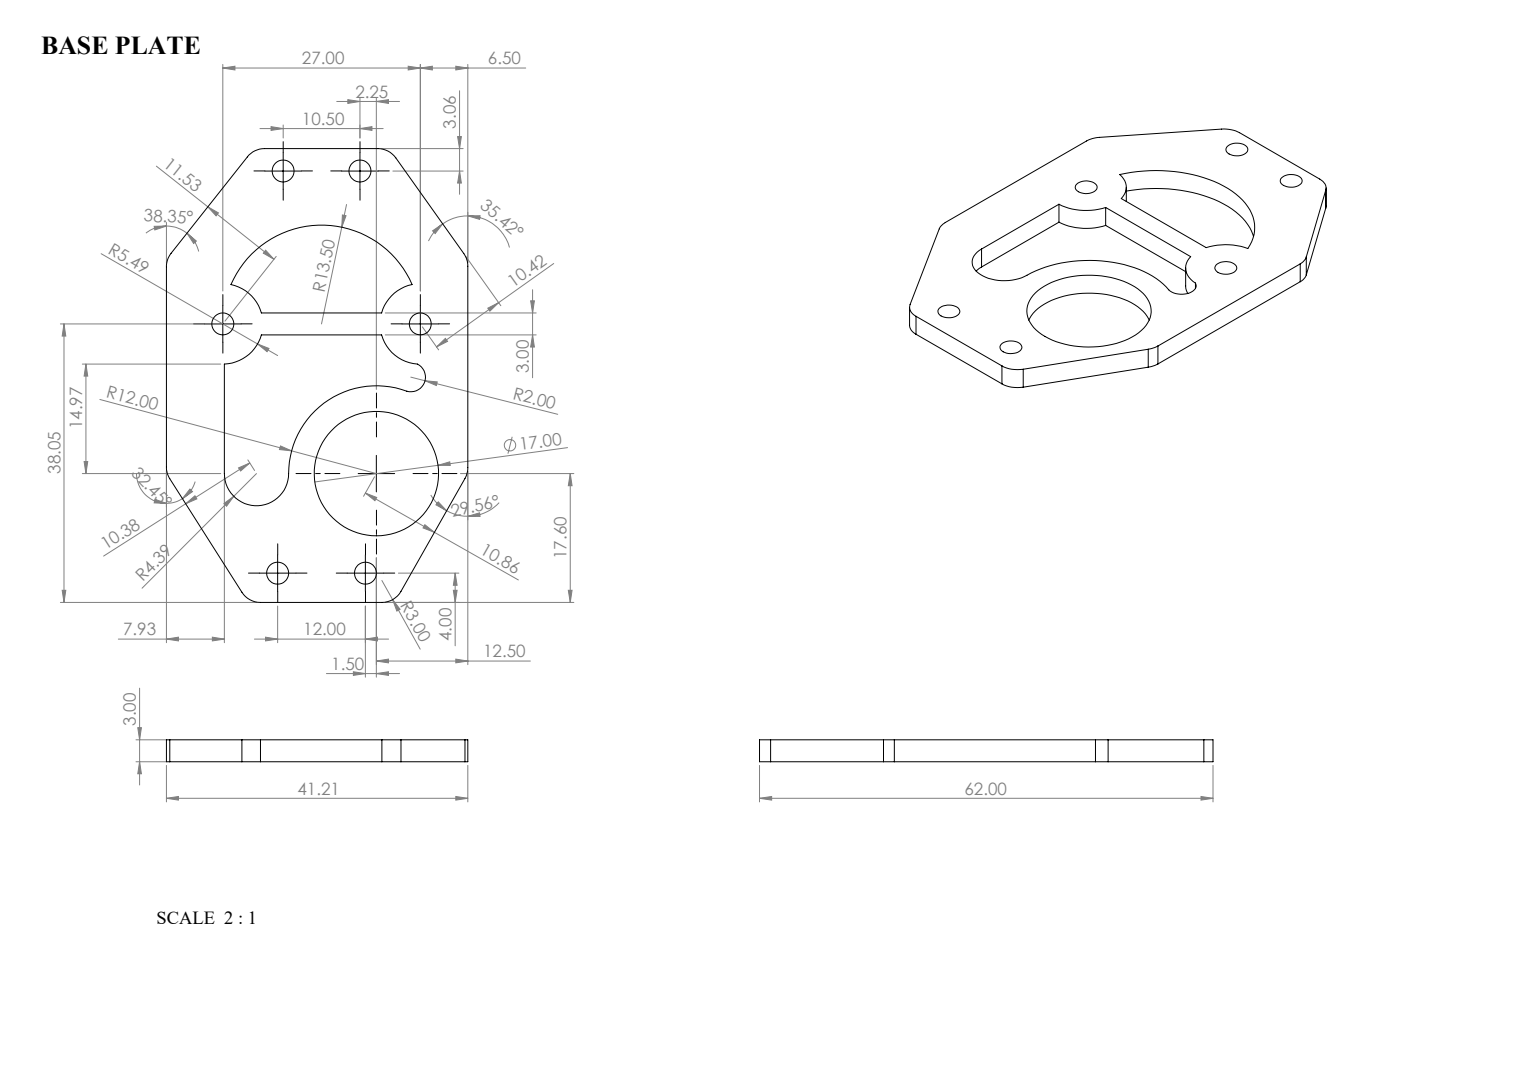
ISO-10303-21;
HEADER;
FILE_DESCRIPTION (('STEP AP214'),
    '1' );
FILE_NAME ('base-plate.step',
    '2026-10-11T23:18:24',
    ( '' ),
    ( '' ),
    'SwSTEP 2.0',
    'SolidWorks 2021',
    '' );
FILE_SCHEMA (( 'AUTOMOTIVE_DESIGN' ));
ENDSEC;

DATA;
#9=FACE_BOUND ( 'NONE', #6807, .T. ) ;
#18=EDGE_LOOP ( 'NONE', ( #222, #3036 ) ) ;
#19=DIRECTION ( 'NONE',  ( -0.000000000000000000, -1.000000000000000000, -0.000000000000000000 ) ) ;
#31=EDGE_CURVE ( 'NONE', #5801, #5272, #8241, .T. ) ;
#45=VERTEX_POINT ( 'NONE', #5075 ) ;
#48=DIRECTION ( 'NONE',  ( 0.000000000000000000, 1.000000000000000000, 0.000000000000000000 ) ) ;
#58=VECTOR ( 'NONE', #8688, 1000.000000000000000 ) ;
#68=VECTOR ( 'NONE', #1053, 1000.000000000000000 ) ;
#77=ORIENTED_EDGE ( 'NONE', *, *, #13230, .T. ) ;
#92=EDGE_CURVE ( 'NONE', #5359, #2558, #6205, .T. ) ;
#98=ORIENTED_EDGE ( 'NONE', *, *, #5069, .T. ) ;
#103=( LENGTH_UNIT ( ) NAMED_UNIT ( * ) SI_UNIT ( .MILLI., .METRE. ) );
#104=DIRECTION ( 'NONE',  ( -0.000000000000000000, -1.000000000000000000, -0.000000000000000000 ) ) ;
#105=CARTESIAN_POINT ( 'NONE',  ( 17.00000000000000711, 0.000000000000000000, 12.57924256039205524 ) ) ;
#107=DIRECTION ( 'NONE',  ( -0.000000000000000000, -1.000000000000000000, -0.000000000000000000 ) ) ;
#111=ADVANCED_FACE ( 'NONE', ( #10454 ), #11355, .F. ) ;
#118=ADVANCED_FACE ( 'NONE', ( #1922 ), #5010, .T. ) ;
#120=CARTESIAN_POINT ( 'NONE',  ( 6.000000000000008882, 3.000000000000000000, 28.50000000000000000 ) ) ;
#124=CARTESIAN_POINT ( 'NONE',  ( -20.74285254778206422, 3.000000000000000000, 14.10762559394868454 ) ) ;
#130=EDGE_CURVE ( 'NONE', #748, #10888, #9495, .T. ) ;
#133=ADVANCED_FACE ( 'NONE', ( #11682 ), #12860, .T. ) ;
#135=ORIENTED_EDGE ( 'NONE', *, *, #11819, .F. ) ;
#147=EDGE_LOOP ( 'NONE', ( #10873, #12283, #1803, #7065 ) ) ;
#148=DIRECTION ( 'NONE',  ( 0.000000000000000000, 1.000000000000000000, 0.000000000000000000 ) ) ;
#150=FACE_BOUND ( 'NONE', #4431, .T. ) ;
#167=DIRECTION ( 'NONE',  ( -1.261435711112880913E-16, -0.000000000000000000, -1.000000000000000000 ) ) ;
#176=CARTESIAN_POINT ( 'NONE',  ( 7.500000000000003553, 0.000000000000000000, 1.399999999999998579 ) ) ;
#180=VERTEX_POINT ( 'NONE', #12788 ) ;
#193=ORIENTED_EDGE ( 'NONE', *, *, #5488, .T. ) ;
#204=ORIENTED_EDGE ( 'NONE', *, *, #9463, .T. ) ;
#208=EDGE_CURVE ( 'NONE', #1513, #12626, #879, .T. ) ;
#222=ORIENTED_EDGE ( 'NONE', *, *, #10239, .T. ) ;
#227=DIRECTION ( 'NONE',  ( 0.000000000000000000, 0.000000000000000000, -1.000000000000000000 ) ) ;
#231=DIRECTION ( 'NONE',  ( -0.000000000000000000, -1.000000000000000000, -0.000000000000000000 ) ) ;
#234=CARTESIAN_POINT ( 'NONE',  ( -20.74285254778206422, 3.000000000000000000, 14.10762559394868454 ) ) ;
#238=ORIENTED_EDGE ( 'NONE', *, *, #208, .T. ) ;
#243=CARTESIAN_POINT ( 'NONE',  ( 7.500000000000003553, 3.000000000000000000, 13.39999999999999858 ) ) ;
#247=CIRCLE ( 'NONE', #1345, 13.50000000000000178 ) ;
#253=AXIS2_PLACEMENT_3D ( 'NONE', #1336, #11952, #4576 ) ;
#265=CARTESIAN_POINT ( 'NONE',  ( -7.798201703419555209, 3.000000000000000000, -30.99999999999999289 ) ) ;
#280=CARTESIAN_POINT ( 'NONE',  ( -21.21140389626389577, 3.000000000000000000, -14.83930531255814955 ) ) ;
#287=ORIENTED_EDGE ( 'NONE', *, *, #2381, .F. ) ;
#308=ORIENTED_EDGE ( 'NONE', *, *, #11057, .T. ) ;
#314=DIRECTION ( 'NONE',  ( -0.000000000000000000, -1.000000000000000000, -0.000000000000000000 ) ) ;
#330=DIRECTION ( 'NONE',  ( -0.000000000000000000, -1.000000000000000000, -0.000000000000000000 ) ) ;
#361=ORIENTED_EDGE ( 'NONE', *, *, #12415, .F. ) ;
#371=DIRECTION ( 'NONE',  ( 0.000000000000000000, 0.000000000000000000, 1.000000000000000000 ) ) ;
#375=VERTEX_POINT ( 'NONE', #9174 ) ;
#381=CARTESIAN_POINT ( 'NONE',  ( 12.21000000000000796, 3.000000000000000000, 0.2208617994340217328 ) ) ;
#383=DIRECTION ( 'NONE',  ( 0.000000000000000000, 0.000000000000000000, -1.000000000000000000 ) ) ;
#415=LINE ( 'NONE', #13021, #10839 ) ;
#435=CARTESIAN_POINT ( 'NONE',  ( 20.00000000000000711, 0.000000000000000000, 12.57924256039204280 ) ) ;
#447=VERTEX_POINT ( 'NONE', #8333 ) ;
#452=CIRCLE ( 'NONE', #7929, 5.499999999999996447 ) ;
#457=LINE ( 'NONE', #7759, #5366 ) ;
#463=CIRCLE ( 'NONE', #3104, 5.486375544325371223 ) ;
#469=ORIENTED_EDGE ( 'NONE', *, *, #9034, .T. ) ;
#470=LINE ( 'NONE', #8726, #4829 ) ;
#471=VECTOR ( 'NONE', #5300, 1000.000000000000000 ) ;
#472=CARTESIAN_POINT ( 'NONE',  ( 12.21000000000000796, 3.000000000000000000, 0.2208617994340217328 ) ) ;
#477=ORIENTED_EDGE ( 'NONE', *, *, #3906, .F. ) ;
#480=UNCERTAINTY_MEASURE_WITH_UNIT (LENGTH_MEASURE( 1.000000000000000082E-05 ), #13297, 'distance_accuracy_value', 'NONE');
#485=ORIENTED_EDGE ( 'NONE', *, *, #6813, .T. ) ;
#497=ORIENTED_EDGE ( 'NONE', *, *, #9087, .T. ) ;
#503=AXIS2_PLACEMENT_3D ( 'NONE', #11418, #6309, #4045 ) ;
#506=CARTESIAN_POINT ( 'NONE',  ( -13.49999999999999645, 0.000000000000000000, -8.549999999999998934 ) ) ;
#526=DIRECTION ( 'NONE',  ( -0.000000000000000000, -1.000000000000000000, -0.000000000000000000 ) ) ;
#528=PRODUCT ( 'base-plate', 'base-plate', '', ( #2121 ) ) ;
#554=DIRECTION ( 'NONE',  ( 1.269138026879196405E-16, 0.000000000000000000, 1.000000000000000000 ) ) ;
#560=AXIS2_PLACEMENT_3D ( 'NONE', #3107, #4208, #10695 ) ;
#577=ORIENTED_EDGE ( 'NONE', *, *, #13185, .F. ) ;
#583=CARTESIAN_POINT ( 'NONE',  ( 8.252687871541644071, 0.000000000000000000, 28.00000000000000000 ) ) ;
#585=DIRECTION ( 'NONE',  ( 0.000000000000000000, 0.000000000000000000, 1.000000000000000000 ) ) ;
#595=EDGE_LOOP ( 'NONE', ( #4853, #1217, #4392, #497, #6612, #11542, #2963, #3783 ) ) ;
#598=CARTESIAN_POINT ( 'NONE',  ( -21.21140389626389222, 0.000000000000000000, 12.49772878833445056 ) ) ;
#607=EDGE_CURVE ( 'NONE', #10071, #5801, #415, .T. ) ;
#621=DIRECTION ( 'NONE',  ( 0.000000000000000000, 0.000000000000000000, 1.000000000000000000 ) ) ;
#634=CARTESIAN_POINT ( 'NONE',  ( -12.38517345876401521, 3.000000000000000000, -12.42191571009144901 ) ) ;
#660=FACE_OUTER_BOUND ( 'NONE', #10677, .T. ) ;
#675=ORIENTED_EDGE ( 'NONE', *, *, #4510, .T. ) ;
#681=EDGE_CURVE ( 'NONE', #2253, #3491, #9506, .T. ) ;
#704=DIRECTION ( 'NONE',  ( 0.000000000000000000, 0.000000000000000000, -1.000000000000000000 ) ) ;
#705=ORIENTED_EDGE ( 'NONE', *, *, #2472, .T. ) ;
#716=CIRCLE ( 'NONE', #13481, 5.486375544325371223 ) ;
#724=PLANE ( 'NONE',  #1129 ) ;
#725=CYLINDRICAL_SURFACE ( 'NONE', #10420, 2.999999999999999112 ) ;
#726=CYLINDRICAL_SURFACE ( 'NONE', #3574, 1.500000000000001332 ) ;
#732=VERTEX_POINT ( 'NONE', #2758 ) ;
#748=VERTEX_POINT ( 'NONE', #8122 ) ;
#779=CARTESIAN_POINT ( 'NONE',  ( -13.49999999999999645, 0.000000000000000000, -7.049999999999998934 ) ) ;
#802=DIRECTION ( 'NONE',  ( -0.000000000000000000, -1.000000000000000000, -0.000000000000000000 ) ) ;
#811=LINE ( 'NONE', #5002, #9521 ) ;
#812=CARTESIAN_POINT ( 'NONE',  ( 7.500000000000003553, 3.000000000000000000, 4.899999999999997691 ) ) ;
#828=ORIENTED_EDGE ( 'NONE', *, *, #11819, .T. ) ;
#833=VERTEX_POINT ( 'NONE', #12065 ) ;
#834=DIRECTION ( 'NONE',  ( 0.000000000000000000, 1.000000000000000000, -0.000000000000000000 ) ) ;
#840=CARTESIAN_POINT ( 'NONE',  ( 8.252687871541644071, 3.000000000000000000, 28.00000000000000000 ) ) ;
#851=PLANE ( 'NONE',  #4516 ) ;
#852=CARTESIAN_POINT ( 'NONE',  ( 8.208497377870827449, 3.000000000000000000, -8.550000000000002487 ) ) ;
#853=CARTESIAN_POINT ( 'NONE',  ( -5.999999999999991118, 0.000000000000000000, 28.50000000000000000 ) ) ;
#867=ORIENTED_EDGE ( 'NONE', *, *, #6355, .F. ) ;
#870=CARTESIAN_POINT ( 'NONE',  ( 7.702138240596505092, 3.000000000000000000, -30.99999999999999289 ) ) ;
#877=ORIENTED_EDGE ( 'NONE', *, *, #6306, .T. ) ;
#879=LINE ( 'NONE', #11884, #4882 ) ;
#889=CARTESIAN_POINT ( 'NONE',  ( -7.798201703419567643, 3.000000000000000000, -27.99999999999999289 ) ) ;
#894=VECTOR ( 'NONE', #3788, 1000.000000000000000 ) ;
#906=DIRECTION ( 'NONE',  ( 0.000000000000000000, 1.000000000000000000, 0.000000000000000000 ) ) ;
#907=DIRECTION ( 'NONE',  ( 0.000000000000000000, 0.000000000000000000, 1.000000000000000000 ) ) ;
#909=EDGE_LOOP ( 'NONE', ( #5022, #6085, #12147, #4456 ) ) ;
#923=CYLINDRICAL_SURFACE ( 'NONE', #4474, 1.499999999999997780 ) ;
#930=VERTEX_POINT ( 'NONE', #3159 ) ;
#932=ORIENTED_EDGE ( 'NONE', *, *, #8564, .T. ) ;
#936=EDGE_CURVE ( 'NONE', #7585, #7204, #7318, .T. ) ;
#950=ORIENTED_EDGE ( 'NONE', *, *, #13438, .T. ) ;
#962=AXIS2_PLACEMENT_3D ( 'NONE', #3139, #7989, #12209 ) ;
#975=CARTESIAN_POINT ( 'NONE',  ( 3.469446951953614189E-15, 0.000000000000000000, -20.55000000000000071 ) ) ;
#983=AXIS2_PLACEMENT_3D ( 'NONE', #6603, #5774, #12198 ) ;
#991=LINE ( 'NONE', #852, #68 ) ;
#996=CIRCLE ( 'NONE', #4722, 1.500000000000001332 ) ;
#998=VECTOR ( 'NONE', #2423, 1000.000000000000114 ) ;
#1005=ORIENTED_EDGE ( 'NONE', *, *, #10913, .T. ) ;
#1042=DIRECTION ( 'NONE',  ( 0.000000000000000000, 1.000000000000000000, -0.000000000000000000 ) ) ;
#1053=DIRECTION ( 'NONE',  ( -0.000000000000000000, -1.000000000000000000, -0.000000000000000000 ) ) ;
#1070=CARTESIAN_POINT ( 'NONE',  ( 5.250000000000000000, 0.000000000000000000, -27.94078293894052578 ) ) ;
#1077=DIRECTION ( 'NONE',  ( -0.000000000000000000, -1.000000000000000000, -0.000000000000000000 ) ) ;
#1080=ADVANCED_FACE ( 'NONE', ( #4393 ), #6669, .T. ) ;
#1081=CARTESIAN_POINT ( 'NONE',  ( 6.000000000000008882, 3.000000000000000000, 25.50000000000000000 ) ) ;
#1087=DIRECTION ( 'NONE',  ( -1.000000000000000000, -0.000000000000000000, -0.000000000000000000 ) ) ;
#1106=FACE_OUTER_BOUND ( 'NONE', #909, .T. ) ;
#1115=EDGE_CURVE ( 'NONE', #3649, #2964, #8630, .T. ) ;
#1122=EDGE_CURVE ( 'NONE', #4943, #748, #7568, .T. ) ;
#1129=AXIS2_PLACEMENT_3D ( 'NONE', #6919, #2580, #11188 ) ;
#1130=CIRCLE ( 'NONE', #7717, 2.000000000000000444 ) ;
#1137=AXIS2_PLACEMENT_3D ( 'NONE', #10482, #6075, #10412 ) ;
#1151=DIRECTION ( 'NONE',  ( -0.000000000000000000, -1.000000000000000000, -0.000000000000000000 ) ) ;
#1163=CARTESIAN_POINT ( 'NONE',  ( -13.49999999999999645, 3.000000000000000000, -7.049999999999998934 ) ) ;
#1166=ORIENTED_EDGE ( 'NONE', *, *, #5988, .F. ) ;
#1167=FACE_BOUND ( 'NONE', #595, .T. ) ;
#1171=AXIS2_PLACEMENT_3D ( 'NONE', #3827, #4855, #8029 ) ;
#1189=AXIS2_PLACEMENT_3D ( 'NONE', #12887, #3430, #7642 ) ;
#1191=CARTESIAN_POINT ( 'NONE',  ( -5.999999999999991118, 3.000000000000000000, 27.00000000000000000 ) ) ;
#1199=DIRECTION ( 'NONE',  ( -0.5795187626277481518, -0.000000000000000000, -0.8149588969772669778 ) ) ;
#1204=ORIENTED_EDGE ( 'NONE', *, *, #12712, .F. ) ;
#1217=ORIENTED_EDGE ( 'NONE', *, *, #12857, .T. ) ;
#1220=DIRECTION ( 'NONE',  ( 0.000000000000000000, 1.000000000000000000, 0.000000000000000000 ) ) ;
#1232=ORIENTED_EDGE ( 'NONE', *, *, #4731, .T. ) ;
#1251=VERTEX_POINT ( 'NONE', #6946 ) ;
#1257=CARTESIAN_POINT ( 'NONE',  ( 13.50000000000000355, 3.000000000000000000, -7.050000000000000711 ) ) ;
#1260=DIRECTION ( 'NONE',  ( 0.000000000000000000, 1.000000000000000000, 0.000000000000000000 ) ) ;
#1280=VERTEX_POINT ( 'NONE', #11075 ) ;
#1283=FACE_OUTER_BOUND ( 'NONE', #7951, .T. ) ;
#1289=CARTESIAN_POINT ( 'NONE',  ( -12.38517345876401521, 0.000000000000000000, -12.42191571009144901 ) ) ;
#1295=CARTESIAN_POINT ( 'NONE',  ( -8.352599575481690408, 3.000000000000000000, 28.00000000000000000 ) ) ;
#1303=ADVANCED_FACE ( 'NONE', ( #6243 ), #5149, .T. ) ;
#1317=LINE ( 'NONE', #9588, #12455 ) ;
#1318=CIRCLE ( 'NONE', #2016, 1.500000000000001332 ) ;
#1320=DIRECTION ( 'NONE',  ( -0.000000000000000000, -1.000000000000000000, -0.000000000000000000 ) ) ;
#1335=DIRECTION ( 'NONE',  ( -0.000000000000000000, -1.000000000000000000, -0.000000000000000000 ) ) ;
#1336=CARTESIAN_POINT ( 'NONE',  ( -13.49999999999999645, 3.000000000000000000, -7.049999999999998934 ) ) ;
#1345=AXIS2_PLACEMENT_3D ( 'NONE', #7820, #3415, #10926 ) ;
#1363=CARTESIAN_POINT ( 'NONE',  ( -7.798201703419567643, 3.000000000000000000, -27.99999999999999289 ) ) ;
#1364=ORIENTED_EDGE ( 'NONE', *, *, #9776, .F. ) ;
#1380=AXIS2_PLACEMENT_3D ( 'NONE', #2769, #13035, #1743 ) ;
#1390=( NAMED_UNIT ( * ) PLANE_ANGLE_UNIT ( ) SI_UNIT ( $, .RADIAN. ) );
#1398=LINE ( 'NONE', #234, #998 ) ;
#1403=ADVANCED_FACE ( 'NONE', ( #3137 ), #3672, .T. ) ;
#1409=VERTEX_POINT ( 'NONE', #12093 ) ;
#1410=DIRECTION ( 'NONE',  ( 0.000000000000000000, 1.000000000000000000, 0.000000000000000000 ) ) ;
#1422=CIRCLE ( 'NONE', #5602, 4.390701948131951582 ) ;
#1454=( NAMED_UNIT ( * ) SI_UNIT ( $, .STERADIAN. ) SOLID_ANGLE_UNIT ( ) );
#1457=PRODUCT_DEFINITION_CONTEXT ( 'detailed design', #12167, 'design' ) ;
#1465=ADVANCED_FACE ( 'NONE', ( #5950 ), #13260, .F. ) ;
#1470=ORIENTED_EDGE ( 'NONE', *, *, #8368, .T. ) ;
#1479=DIRECTION ( 'NONE',  ( -0.000000000000000000, -1.000000000000000000, -0.000000000000000000 ) ) ;
#1489=DIRECTION ( 'NONE',  ( -0.6204948238377417935, -0.000000000000000000, 0.7842105416216806901 ) ) ;
#1503=ADVANCED_FACE ( 'NONE', ( #2924 ), #725, .T. ) ;
#1505=CYLINDRICAL_SURFACE ( 'NONE', #12322, 1.499999999999999556 ) ;
#1507=CARTESIAN_POINT ( 'NONE',  ( 20.00000000000000711, 3.000000000000000000, 12.57924256039204280 ) ) ;
#1513=VERTEX_POINT ( 'NONE', #6993 ) ;
#1515=VERTEX_POINT ( 'NONE', #7874 ) ;
#1532=CYLINDRICAL_SURFACE ( 'NONE', #6265, 1.500000000000001332 ) ;
#1549=FACE_BOUND ( 'NONE', #2100, .T. ) ;
#1550=CARTESIAN_POINT ( 'NONE',  ( 5.250000000000000000, 3.000000000000000000, -27.94078293894052578 ) ) ;
#1559=DIRECTION ( 'NONE',  ( 0.000000000000000000, 1.000000000000000000, 0.000000000000000000 ) ) ;
#1567=ORIENTED_EDGE ( 'NONE', *, *, #11702, .F. ) ;
#1600=CIRCLE ( 'NONE', #7756, 2.999999999999999112 ) ;
#1612=AXIS2_PLACEMENT_3D ( 'NONE', #5175, #8323, #10405 ) ;
#1613=AXIS2_PLACEMENT_3D ( 'NONE', #13583, #19, #10548 ) ;
#1614=DIRECTION ( 'NONE',  ( 0.000000000000000000, 0.000000000000000000, -1.000000000000000000 ) ) ;
#1622=FACE_BOUND ( 'NONE', #4217, .T. ) ;
#1626=AXIS2_PLACEMENT_3D ( 'NONE', #11875, #9668, #5531 ) ;
#1629=ADVANCED_FACE ( 'NONE', ( #3784 ), #8372, .F. ) ;
#1631=EDGE_CURVE ( 'NONE', #8075, #1251, #9534, .T. ) ;
#1642=DIRECTION ( 'NONE',  ( -1.000000000000000000, -0.000000000000000000, 1.055752450943286591E-16 ) ) ;
#1664=AXIS2_PLACEMENT_3D ( 'NONE', #2975, #7186, #11378 ) ;
#1668=VERTEX_POINT ( 'NONE', #3475 ) ;
#1678=FACE_OUTER_BOUND ( 'NONE', #5525, .T. ) ;
#1684=PRODUCT_DEFINITION_FORMATION_WITH_SPECIFIED_SOURCE ( 'ANY', '', #528, .NOT_KNOWN. ) ;
#1694=CARTESIAN_POINT ( 'NONE',  ( 3.469446951953614189E-15, 3.000000000000000000, -7.049999999999999822 ) ) ;
#1700=CARTESIAN_POINT ( 'NONE',  ( -21.21140389626389577, 3.000000000000000000, -14.83930531255815133 ) ) ;
#1714=VERTEX_POINT ( 'NONE', #4380 ) ;
#1729=UNCERTAINTY_MEASURE_WITH_UNIT (LENGTH_MEASURE( 1.000000000000000082E-05 ), #103, 'distance_accuracy_value', 'NONE');
#1736=VERTEX_POINT ( 'NONE', #3413 ) ;
#1742=VERTEX_POINT ( 'NONE', #5543 ) ;
#1743=DIRECTION ( 'NONE',  ( 0.000000000000000000, 0.000000000000000000, -1.000000000000000000 ) ) ;
#1755=DIRECTION ( 'NONE',  ( 0.000000000000000000, 0.000000000000000000, 1.000000000000000000 ) ) ;
#1802=CIRCLE ( 'NONE', #253, 1.499999999999998668 ) ;
#1803=ORIENTED_EDGE ( 'NONE', *, *, #11372, .F. ) ;
#1806=FACE_OUTER_BOUND ( 'NONE', #13472, .T. ) ;
#1811=AXIS2_PLACEMENT_3D ( 'NONE', #10518, #1077, #13417 ) ;
#1813=AXIS2_PLACEMENT_3D ( 'NONE', #12705, #3315, #5319 ) ;
#1829=EDGE_CURVE ( 'NONE', #5704, #11250, #10986, .T. ) ;
#1831=CARTESIAN_POINT ( 'NONE',  ( -13.49999999999999645, 3.000000000000000000, -7.049999999999998934 ) ) ;
#1834=ORIENTED_EDGE ( 'NONE', *, *, #10278, .T. ) ;
#1838=VERTEX_POINT ( 'NONE', #598 ) ;
#1845=DIRECTION ( 'NONE',  ( 0.000000000000000000, 0.000000000000000000, 1.000000000000000000 ) ) ;
#1859=AXIS2_PLACEMENT_3D ( 'NONE', #3543, #10859, #2450 ) ;
#1881=ADVANCED_FACE ( 'NONE', ( #10159 ), #10089, .T. ) ;
#1910=EDGE_CURVE ( 'NONE', #1668, #1714, #12249, .T. ) ;
#1919=CARTESIAN_POINT ( 'NONE',  ( -13.28140389626389783, 0.000000000000000000, 13.39999999999999858 ) ) ;
#1922=FACE_OUTER_BOUND ( 'NONE', #3038, .T. ) ;
#1926=DIRECTION ( 'NONE',  ( -0.000000000000000000, -1.000000000000000000, -0.000000000000000000 ) ) ;
#1928=DIRECTION ( 'NONE',  ( -0.000000000000000000, -1.000000000000000000, -0.000000000000000000 ) ) ;
#1934=ORIENTED_EDGE ( 'NONE', *, *, #3335, .T. ) ;
#1957=DIRECTION ( 'NONE',  ( -0.000000000000000000, -1.000000000000000000, -0.000000000000000000 ) ) ;
#1969=EDGE_CURVE ( 'NONE', #8365, #12893, #8158, .T. ) ;
#1977=VECTOR ( 'NONE', #1151, 1000.000000000000000 ) ;
#1978=DIRECTION ( 'NONE',  ( -0.000000000000000000, -1.000000000000000000, -0.000000000000000000 ) ) ;
#1980=ORIENTED_EDGE ( 'NONE', *, *, #13096, .F. ) ;
#1989=DIRECTION ( 'NONE',  ( -0.000000000000000000, -1.000000000000000000, -0.000000000000000000 ) ) ;
#2000=ORIENTED_EDGE ( 'NONE', *, *, #2363, .T. ) ;
#2002=VECTOR ( 'NONE', #2219, 1000.000000000000000 ) ;
#2005=CIRCLE ( 'NONE', #10360, 5.486375544325371223 ) ;
#2008=LINE ( 'NONE', #6202, #3327 ) ;
#2016=AXIS2_PLACEMENT_3D ( 'NONE', #3607, #2438, #8760 ) ;
#2022=EDGE_CURVE ( 'NONE', #4834, #8240, #9329, .T. ) ;
#2029=VERTEX_POINT ( 'NONE', #13547 ) ;
#2033=VERTEX_POINT ( 'NONE', #12583 ) ;
#2034=AXIS2_PLACEMENT_3D ( 'NONE', #3071, #7284, #11481 ) ;
#2046=AXIS2_PLACEMENT_3D ( 'NONE', #3810, #13115, #585 ) ;
#2047=EDGE_CURVE ( 'NONE', #5599, #2682, #12427, .T. ) ;
#2051=ORIENTED_EDGE ( 'NONE', *, *, #3303, .F. ) ;
#2060=EDGE_CURVE ( 'NONE', #930, #13159, #3377, .T. ) ;
#2073=FACE_BOUND ( 'NONE', #18, .T. ) ;
#2100=EDGE_LOOP ( 'NONE', ( #2226, #8679 ) ) ;
#2103=AXIS2_PLACEMENT_3D ( 'NONE', #9001, #13218, #13089 ) ;
#2107=DIRECTION ( 'NONE',  ( 0.8438162171727213723, 0.000000000000000000, -0.5366322685380732205 ) ) ;
#2108=CARTESIAN_POINT ( 'NONE',  ( 12.37962962962963864, 3.000000000000000000, -12.43467921358330663 ) ) ;
#2121=PRODUCT_CONTEXT ( 'NONE', #8884, 'mechanical' ) ;
#2122=DIRECTION ( 'NONE',  ( -0.000000000000000000, -1.000000000000000000, -0.000000000000000000 ) ) ;
#2137=CARTESIAN_POINT ( 'NONE',  ( 13.50000000000000355, 0.000000000000000000, -5.550000000000001599 ) ) ;
#2145=EDGE_CURVE ( 'NONE', #6080, #1742, #5459, .T. ) ;
#2150=EDGE_CURVE ( 'NONE', #3649, #5599, #3256, .T. ) ;
#2151=PLANE ( 'NONE',  #2311 ) ;
#2153=CARTESIAN_POINT ( 'NONE',  ( 13.50000000000000355, 0.000000000000000000, -7.050000000000000711 ) ) ;
#2154=LINE ( 'NONE', #5315, #7062 ) ;
#2163=EDGE_CURVE ( 'NONE', #10097, #12683, #11083, .T. ) ;
#2168=DIRECTION ( 'NONE',  ( 0.000000000000000000, 0.000000000000000000, 1.000000000000000000 ) ) ;
#2176=ORIENTED_EDGE ( 'NONE', *, *, #10005, .T. ) ;
#2190=ORIENTED_EDGE ( 'NONE', *, *, #6830, .T. ) ;
#2193=CARTESIAN_POINT ( 'NONE',  ( -8.352599575481690408, 3.000000000000000000, 30.99999999999999289 ) ) ;
#2212=VERTEX_POINT ( 'NONE', #435 ) ;
#2218=DIRECTION ( 'NONE',  ( 0.000000000000000000, 0.000000000000000000, 1.000000000000000000 ) ) ;
#2219=DIRECTION ( 'NONE',  ( -0.000000000000000000, -1.000000000000000000, -0.000000000000000000 ) ) ;
#2226=ORIENTED_EDGE ( 'NONE', *, *, #10278, .F. ) ;
#2233=PLANE ( 'NONE',  #13273 ) ;
#2253=VERTEX_POINT ( 'NONE', #506 ) ;
#2258=VECTOR ( 'NONE', #7072, 1000.000000000000000 ) ;
#2282=CIRCLE ( 'NONE', #10203, 1.500000000000001332 ) ;
#2283=EDGE_CURVE ( 'NONE', #10892, #10734, #2720, .T. ) ;
#2294=ORIENTED_EDGE ( 'NONE', *, *, #8948, .F. ) ;
#2304=EDGE_CURVE ( 'NONE', #11250, #6484, #11758, .T. ) ;
#2309=CARTESIAN_POINT ( 'NONE',  ( -8.890701948131944476, 0.000000000000000000, 13.39999999999999858 ) ) ;
#2311=AXIS2_PLACEMENT_3D ( 'NONE', #5383, #11724, #2356 ) ;
#2314=CARTESIAN_POINT ( 'NONE',  ( -8.222660081691577361, 0.000000000000000000, -8.549999999999998934 ) ) ;
#2316=ORIENTED_EDGE ( 'NONE', *, *, #6450, .F. ) ;
#2337=ORIENTED_EDGE ( 'NONE', *, *, #9364, .F. ) ;
#2349=VERTEX_POINT ( 'NONE', #12371 ) ;
#2356=DIRECTION ( 'NONE',  ( -1.000000000000000000, 0.000000000000000000, -0.000000000000000000 ) ) ;
#2358=LINE ( 'NONE', #5447, #6645 ) ;
#2363=EDGE_CURVE ( 'NONE', #375, #2349, #3043, .T. ) ;
#2370=VERTEX_POINT ( 'NONE', #6087 ) ;
#2371=ORIENTED_EDGE ( 'NONE', *, *, #10453, .F. ) ;
#2381=EDGE_CURVE ( 'NONE', #3023, #4625, #13086, .T. ) ;
#2382=CARTESIAN_POINT ( 'NONE',  ( 8.252687871541644071, 3.000000000000000000, 28.00000000000000000 ) ) ;
#2386=CYLINDRICAL_SURFACE ( 'NONE', #12106, 4.390701948131951582 ) ;
#2396=ORIENTED_EDGE ( 'NONE', *, *, #7136, .T. ) ;
#2397=VERTEX_POINT ( 'NONE', #12564 ) ;
#2400=DIRECTION ( 'NONE',  ( -0.000000000000000000, -1.000000000000000000, -0.000000000000000000 ) ) ;
#2404=PLANE ( 'NONE',  #983 ) ;
#2408=ORIENTED_EDGE ( 'NONE', *, *, #9087, .F. ) ;
#2417=CIRCLE ( 'NONE', #10989, 5.499999999999996447 ) ;
#2418=DIRECTION ( 'NONE',  ( -0.000000000000000000, -1.000000000000000000, -0.000000000000000000 ) ) ;
#2420=AXIS2_PLACEMENT_3D ( 'NONE', #2918, #9592, #5385 ) ;
#2423=DIRECTION ( 'NONE',  ( 0.5366322685380732205, 0.000000000000000000, 0.8438162171727212613 ) ) ;
#2425=CARTESIAN_POINT ( 'NONE',  ( 10.14701493152832512, 0.000000000000000000, -29.73855628788322747 ) ) ;
#2428=CIRCLE ( 'NONE', #2860, 1.500000000000001332 ) ;
#2438=DIRECTION ( 'NONE',  ( 0.000000000000000000, 1.000000000000000000, 0.000000000000000000 ) ) ;
#2442=EDGE_LOOP ( 'NONE', ( #1232, #11128, #3557, #3779 ) ) ;
#2443=ORIENTED_EDGE ( 'NONE', *, *, #12580, .F. ) ;
#2445=AXIS2_PLACEMENT_3D ( 'NONE', #9870, #7615, #6573 ) ;
#2450=DIRECTION ( 'NONE',  ( 1.000000000000000000, 0.000000000000000000, -0.000000000000000000 ) ) ;
#2454=LINE ( 'NONE', #812, #9672 ) ;
#2463=ORIENTED_EDGE ( 'NONE', *, *, #1910, .T. ) ;
#2464=CARTESIAN_POINT ( 'NONE',  ( 12.37962962962963864, 3.000000000000000000, -12.43467921358330663 ) ) ;
#2472=EDGE_CURVE ( 'NONE', #3370, #11639, #1317, .T. ) ;
#2482=CARTESIAN_POINT ( 'NONE',  ( -13.49999999999999645, 0.000000000000000000, -7.049999999999998934 ) ) ;
#2487=CARTESIAN_POINT ( 'NONE',  ( -8.352599575481690408, 0.000000000000000000, 30.99999999999999289 ) ) ;
#2489=FILL_AREA_STYLE ('',( #4555 ) ) ;
#2490=CIRCLE ( 'NONE', #1626, 1.499999999999998668 ) ;
#2492=DIRECTION ( 'NONE',  ( 0.000000000000000000, 1.000000000000000000, -0.000000000000000000 ) ) ;
#2509=CIRCLE ( 'NONE', #8877, 12.00000000000000000 ) ;
#2515=ORIENTED_EDGE ( 'NONE', *, *, #2163, .T. ) ;
#2517=ORIENTED_EDGE ( 'NONE', *, *, #6588, .T. ) ;
#2527=STYLED_ITEM ( 'NONE', ( #7719 ), #3745 ) ;
#2529=CIRCLE ( 'NONE', #8674, 1.500000000000001332 ) ;
#2530=ADVANCED_FACE ( 'NONE', ( #11596 ), #2151, .F. ) ;
#2542=DIRECTION ( 'NONE',  ( -0.000000000000000000, -1.000000000000000000, -0.000000000000000000 ) ) ;
#2558=VERTEX_POINT ( 'NONE', #10693 ) ;
#2580=DIRECTION ( 'NONE',  ( 0.000000000000000000, -1.000000000000000000, 0.000000000000000000 ) ) ;
#2614=ORIENTED_EDGE ( 'NONE', *, *, #2304, .T. ) ;
#2623=AXIS2_PLACEMENT_3D ( 'NONE', #3492, #10800, #11910 ) ;
#2629=ORIENTED_EDGE ( 'NONE', *, *, #7346, .F. ) ;
#2634=CARTESIAN_POINT ( 'NONE',  ( -8.890701948131944476, 3.000000000000000000, 13.39999999999999858 ) ) ;
#2655=CARTESIAN_POINT ( 'NONE',  ( -20.56403552112892896, 3.000000000000000000, -16.70078978407140013 ) ) ;
#2660=AXIS2_PLACEMENT_3D ( 'NONE', #9121, #8907, #11125 ) ;
#2661=ORIENTED_EDGE ( 'NONE', *, *, #2022, .T. ) ;
#2682=VERTEX_POINT ( 'NONE', #2487 ) ;
#2684=ORIENTED_EDGE ( 'NONE', *, *, #2047, .T. ) ;
#2696=ORIENTED_EDGE ( 'NONE', *, *, #3385, .T. ) ;
#2707=DIRECTION ( 'NONE',  ( 0.000000000000000000, 0.000000000000000000, -1.000000000000000000 ) ) ;
#2712=FACE_BOUND ( 'NONE', #10036, .T. ) ;
#2720=CIRCLE ( 'NONE', #5368, 13.50000000000000178 ) ;
#2734=VECTOR ( 'NONE', #1978, 1000.000000000000000 ) ;
#2744=AXIS2_PLACEMENT_3D ( 'NONE', #13045, #3525, #3664 ) ;
#2752=EDGE_CURVE ( 'NONE', #4632, #5256, #3472, .T. ) ;
#2758=CARTESIAN_POINT ( 'NONE',  ( -7.798201703419555209, 0.000000000000000000, -30.99999999999999289 ) ) ;
#2760=CARTESIAN_POINT ( 'NONE',  ( 7.500000000000003553, 0.000000000000000000, 13.39999999999999858 ) ) ;
#2769=CARTESIAN_POINT ( 'NONE',  ( -13.49999999999999645, 3.000000000000000000, -7.049999999999998934 ) ) ;
#2789=ORIENTED_EDGE ( 'NONE', *, *, #1829, .F. ) ;
#2800=CARTESIAN_POINT ( 'NONE',  ( 19.44487669093179605, 3.000000000000000000, -16.66326752702930847 ) ) ;
#2815=LINE ( 'NONE', #11015, #5780 ) ;
#2835=ORIENTED_EDGE ( 'NONE', *, *, #9258, .T. ) ;
#2860=AXIS2_PLACEMENT_3D ( 'NONE', #11334, #13183, #13336 ) ;
#2901=FACE_OUTER_BOUND ( 'NONE', #7066, .T. ) ;
#2908=ADVANCED_FACE ( 'NONE', ( #12743, #1167, #6393, #150, #4399, #8460, #9, #12685, #2073, #5294 ), #7571, .T. ) ;
#2912=CARTESIAN_POINT ( 'NONE',  ( -20.74285254778206067, 3.000000000000000000, 14.10762559394868099 ) ) ;
#2914=CARTESIAN_POINT ( 'NONE',  ( -5.999999999999991118, 0.000000000000000000, 27.00000000000000000 ) ) ;
#2918=CARTESIAN_POINT ( 'NONE',  ( -13.28140389626389783, 3.000000000000000000, 13.39999999999999858 ) ) ;
#2924=FACE_OUTER_BOUND ( 'NONE', #13436, .T. ) ;
#2932=DIRECTION ( 'NONE',  ( -0.000000000000000000, -1.000000000000000000, -0.000000000000000000 ) ) ;
#2940=DIRECTION ( 'NONE',  ( -0.000000000000000000, -1.000000000000000000, -0.000000000000000000 ) ) ;
#2963=ORIENTED_EDGE ( 'NONE', *, *, #13274, .T. ) ;
#2964=VERTEX_POINT ( 'NONE', #2193 ) ;
#2975=CARTESIAN_POINT ( 'NONE',  ( 17.00000000000000711, 3.000000000000000000, 12.57924256039205524 ) ) ;
#2989=CARTESIAN_POINT ( 'NONE',  ( -20.74285254778206422, 0.000000000000000000, 14.10762559394868454 ) ) ;
#2991=LINE ( 'NONE', #11395, #5277 ) ;
#3009=DIRECTION ( 'NONE',  ( 0.000000000000000000, 0.000000000000000000, -1.000000000000000000 ) ) ;
#3021=CARTESIAN_POINT ( 'NONE',  ( 13.50000000000000355, 3.000000000000000000, -5.550000000000001599 ) ) ;
#3023=VERTEX_POINT ( 'NONE', #3161 ) ;
#3028=PRODUCT_DEFINITION ( 'UNKNOWN', '', #1684, #1457 ) ;
#3035=CARTESIAN_POINT ( 'NONE',  ( -5.999999999999991118, 0.000000000000000000, 27.00000000000000000 ) ) ;
#3036=ORIENTED_EDGE ( 'NONE', *, *, #10962, .T. ) ;
#3038=EDGE_LOOP ( 'NONE', ( #11382, #2337, #10364, #5538 ) ) ;
#3041=EDGE_CURVE ( 'NONE', #2033, #12313, #8992, .T. ) ;
#3043=LINE ( 'NONE', #2912, #3168 ) ;
#3047=DIRECTION ( 'NONE',  ( 0.5366322685380732205, 0.000000000000000000, 0.8438162171727212613 ) ) ;
#3048=CARTESIAN_POINT ( 'NONE',  ( 7.702138240596516638, 3.000000000000000000, -27.99999999999999289 ) ) ;
#3059=ADVANCED_FACE ( 'NONE', ( #6601 ), #1505, .F. ) ;
#3062=DIRECTION ( 'NONE',  ( 0.000000000000000000, 0.000000000000000000, 1.000000000000000000 ) ) ;
#3067=DIRECTION ( 'NONE',  ( 0.000000000000000000, 1.000000000000000000, -0.000000000000000000 ) ) ;
#3069=EDGE_LOOP ( 'NONE', ( #8602, #1980, #6687, #5840 ) ) ;
#3070=EDGE_CURVE ( 'NONE', #2033, #8075, #470, .T. ) ;
#3071=CARTESIAN_POINT ( 'NONE',  ( -5.250000000000000000, 3.000000000000000000, -27.94078293894052578 ) ) ;
#3082=AXIS2_PLACEMENT_3D ( 'NONE', #3360, #3227, #6536 ) ;
#3095=CARTESIAN_POINT ( 'NONE',  ( 3.469446951953614189E-15, 3.000000000000000000, -20.55000000000000071 ) ) ;
#3098=ADVANCED_FACE ( 'NONE', ( #5491 ), #9699, .T. ) ;
#3104=AXIS2_PLACEMENT_3D ( 'NONE', #8100, #11272, #1845 ) ;
#3107=CARTESIAN_POINT ( 'NONE',  ( -21.21140389626389577, 3.000000000000000000, -14.83930531255815133 ) ) ;
#3108=DIRECTION ( 'NONE',  ( -0.000000000000000000, -1.000000000000000000, -0.000000000000000000 ) ) ;
#3109=DIRECTION ( 'NONE',  ( 0.000000000000000000, 1.000000000000000000, 0.000000000000000000 ) ) ;
#3122=AXIS2_PLACEMENT_3D ( 'NONE', #11280, #12531, #7157 ) ;
#3123=AXIS2_PLACEMENT_3D ( 'NONE', #9612, #7674, #383 ) ;
#3131=VECTOR ( 'NONE', #5384, 1000.000000000000000 ) ;
#3137=FACE_OUTER_BOUND ( 'NONE', #11415, .T. ) ;
#3139=CARTESIAN_POINT ( 'NONE',  ( 5.250000000000000000, 3.000000000000000000, -27.94078293894052578 ) ) ;
#3140=PRODUCT_DEFINITION_SHAPE ( 'NONE', 'NONE',  #3028 ) ;
#3143=CARTESIAN_POINT ( 'NONE',  ( 20.00000000000000711, 3.000000000000000000, 12.57924256039204280 ) ) ;
#3156=ORIENTED_EDGE ( 'NONE', *, *, #7047, .T. ) ;
#3159=CARTESIAN_POINT ( 'NONE',  ( 10.14701493152832512, 0.000000000000000000, -29.73855628788322747 ) ) ;
#3161=CARTESIAN_POINT ( 'NONE',  ( 5.250000000000000000, 3.000000000000000000, -26.44078293894052578 ) ) ;
#3168=VECTOR ( 'NONE', #5041, 1000.000000000000000 ) ;
#3176=VECTOR ( 'NONE', #8703, 1000.000000000000000 ) ;
#3178=CIRCLE ( 'NONE', #6255, 2.999999999999999112 ) ;
#3188=MECHANICAL_DESIGN_GEOMETRIC_PRESENTATION_REPRESENTATION('',(#2527),#4076);
#3197=ORIENTED_EDGE ( 'NONE', *, *, #3974, .F. ) ;
#3205=DIRECTION ( 'NONE',  ( 0.000000000000000000, 0.000000000000000000, 1.000000000000000000 ) ) ;
#3206=CARTESIAN_POINT ( 'NONE',  ( 17.00000000000000355, 3.000000000000000000, -14.92471123914605435 ) ) ;
#3219=CARTESIAN_POINT ( 'NONE',  ( -8.222660081691577361, 3.000000000000000000, -5.549999999999999822 ) ) ;
#3227=DIRECTION ( 'NONE',  ( 0.000000000000000000, -1.000000000000000000, 0.000000000000000000 ) ) ;
#3243=ORIENTED_EDGE ( 'NONE', *, *, #9776, .T. ) ;
#3246=DIRECTION ( 'NONE',  ( 0.000000000000000000, 1.000000000000000000, 0.000000000000000000 ) ) ;
#3256=LINE ( 'NONE', #4433, #13060 ) ;
#3260=CARTESIAN_POINT ( 'NONE',  ( 10.86210944460165528, 0.000000000000000000, 29.48017534571043541 ) ) ;
#3289=DIRECTION ( 'NONE',  ( 0.000000000000000000, 1.000000000000000000, 0.000000000000000000 ) ) ;
#3294=AXIS2_PLACEMENT_3D ( 'NONE', #9701, #10681, #10539 ) ;
#3296=EDGE_LOOP ( 'NONE', ( #6577, #5303, #675, #4112 ) ) ;
#3303=EDGE_CURVE ( 'NONE', #5027, #3357, #5081, .T. ) ;
#3315=DIRECTION ( 'NONE',  ( -0.000000000000000000, -1.000000000000000000, -0.000000000000000000 ) ) ;
#3319=CARTESIAN_POINT ( 'NONE',  ( 5.250000000000000000, 3.000000000000000000, -29.44078293894052933 ) ) ;
#3327=VECTOR ( 'NONE', #12359, 1000.000000000000000 ) ;
#3330=CARTESIAN_POINT ( 'NONE',  ( -8.222660081691577361, 3.000000000000000000, -8.549999999999998934 ) ) ;
#3335=EDGE_CURVE ( 'NONE', #12461, #4201, #6313, .T. ) ;
#3356=AXIS2_PLACEMENT_3D ( 'NONE', #12930, #7625, #9752 ) ;
#3357=VERTEX_POINT ( 'NONE', #5351 ) ;
#3360=CARTESIAN_POINT ( 'NONE',  ( -7.798201703419567643, 0.000000000000000000, -27.99999999999999289 ) ) ;
#3370=VERTEX_POINT ( 'NONE', #3143 ) ;
#3377=CIRCLE ( 'NONE', #4701, 2.999999999999999112 ) ;
#3378=AXIS2_PLACEMENT_3D ( 'NONE', #7576, #6542, #6474 ) ;
#3381=DIRECTION ( 'NONE',  ( 0.000000000000000000, 0.000000000000000000, 1.000000000000000000 ) ) ;
#3382=FACE_OUTER_BOUND ( 'NONE', #7189, .T. ) ;
#3383=CYLINDRICAL_SURFACE ( 'NONE', #7697, 8.500000000000000000 ) ;
#3385=EDGE_CURVE ( 'NONE', #13469, #45, #8507, .T. ) ;
#3391=EDGE_LOOP ( 'NONE', ( #12627, #12308, #1470, #238 ) ) ;
#3399=AXIS2_PLACEMENT_3D ( 'NONE', #7040, #13239, #5796 ) ;
#3402=DIRECTION ( 'NONE',  ( 0.000000000000000000, 0.000000000000000000, 1.000000000000000000 ) ) ;
#3408=VECTOR ( 'NONE', #9978, 1000.000000000000000 ) ;
#3409=ORIENTED_EDGE ( 'NONE', *, *, #11372, .T. ) ;
#3413=CARTESIAN_POINT ( 'NONE',  ( -10.15083332828461771, 3.000000000000000000, -29.86148447151320795 ) ) ;
#3414=FACE_OUTER_BOUND ( 'NONE', #7967, .T. ) ;
#3415=DIRECTION ( 'NONE',  ( 0.000000000000000000, 1.000000000000000000, 0.000000000000000000 ) ) ;
#3417=CARTESIAN_POINT ( 'NONE',  ( -7.798201703419567643, 0.000000000000000000, -27.99999999999999289 ) ) ;
#3422=EDGE_LOOP ( 'NONE', ( #1567, #287 ) ) ;
#3430=DIRECTION ( 'NONE',  ( 0.000000000000000000, 1.000000000000000000, 0.000000000000000000 ) ) ;
#3456=EDGE_LOOP ( 'NONE', ( #11445, #7984, #6228, #8705 ) ) ;
#3462=DIRECTION ( 'NONE',  ( 0.000000000000000000, 0.000000000000000000, 1.000000000000000000 ) ) ;
#3470=ORIENTED_EDGE ( 'NONE', *, *, #9513, .F. ) ;
#3472=CIRCLE ( 'NONE', #8104, 2.999999999999999112 ) ;
#3475=CARTESIAN_POINT ( 'NONE',  ( -21.21140389626389577, 3.000000000000000000, -14.83930531255814955 ) ) ;
#3491=VERTEX_POINT ( 'NONE', #12232 ) ;
#3492=CARTESIAN_POINT ( 'NONE',  ( 7.500000000000003553, 3.000000000000000000, 13.39999999999999858 ) ) ;
#3510=DIRECTION ( 'NONE',  ( 0.000000000000000000, 0.000000000000000000, 1.000000000000000000 ) ) ;
#3518=LINE ( 'NONE', #2425, #5115 ) ;
#3520=ORIENTED_EDGE ( 'NONE', *, *, #13438, .F. ) ;
#3521=VECTOR ( 'NONE', #5004, 1000.000000000000000 ) ;
#3525=DIRECTION ( 'NONE',  ( -0.000000000000000000, -1.000000000000000000, -0.000000000000000000 ) ) ;
#3540=VECTOR ( 'NONE', #10293, 1000.000000000000000 ) ;
#3543=CARTESIAN_POINT ( 'NONE',  ( -7.798201703419555209, 3.000000000000000000, -30.99999999999999289 ) ) ;
#3544=ADVANCED_FACE ( 'NONE', ( #1283 ), #5545, .T. ) ;
#3552=CARTESIAN_POINT ( 'NONE',  ( 3.469446951953614189E-15, 3.000000000000000000, -7.049999999999999822 ) ) ;
#3557=ORIENTED_EDGE ( 'NONE', *, *, #130, .F. ) ;
#3560=AXIS2_PLACEMENT_3D ( 'NONE', #2482, #9842, #6551 ) ;
#3569=CARTESIAN_POINT ( 'NONE',  ( 13.11311062740304401, 3.000000000000000000, -1.563624455674628377 ) ) ;
#3572=FACE_OUTER_BOUND ( 'NONE', #8262, .T. ) ;
#3574=AXIS2_PLACEMENT_3D ( 'NONE', #1550, #12166, #5741 ) ;
#3607=CARTESIAN_POINT ( 'NONE',  ( 6.000000000000008882, 0.000000000000000000, 27.00000000000000000 ) ) ;
#3613=ADVANCED_FACE ( 'NONE', ( #3414 ), #2386, .F. ) ;
#3622=AXIS2_PLACEMENT_3D ( 'NONE', #7393, #12759, #227 ) ;
#3634=EDGE_CURVE ( 'NONE', #10193, #7606, #6808, .T. ) ;
#3649=VERTEX_POINT ( 'NONE', #7257 ) ;
#3664=DIRECTION ( 'NONE',  ( 0.000000000000000000, 0.000000000000000000, 1.000000000000000000 ) ) ;
#3672=PLANE ( 'NONE',  #9747 ) ;
#3683=ADVANCED_FACE ( 'NONE', ( #5117 ), #7197, .T. ) ;
#3686=LINE ( 'NONE', #6789, #13503 ) ;
#3689=ORIENTED_EDGE ( 'NONE', *, *, #7911, .T. ) ;
#3692=DIRECTION ( 'NONE',  ( 0.000000000000000000, 0.000000000000000000, 1.000000000000000000 ) ) ;
#3702=VERTEX_POINT ( 'NONE', #853 ) ;
#3707=ORIENTED_EDGE ( 'NONE', *, *, #6449, .F. ) ;
#3733=ADVANCED_FACE ( 'NONE', ( #3940 ), #8143, .T. ) ;
#3745=ADVANCED_BREP_SHAPE_REPRESENTATION ( '', ( #8567, #10007 ), #10678 ) ;
#3763=ORIENTED_EDGE ( 'NONE', *, *, #10239, .F. ) ;
#3768=CIRCLE ( 'NONE', #1137, 12.00000000000000000 ) ;
#3779=ORIENTED_EDGE ( 'NONE', *, *, #1122, .F. ) ;
#3783=ORIENTED_EDGE ( 'NONE', *, *, #10040, .T. ) ;
#3784=FACE_OUTER_BOUND ( 'NONE', #6403, .T. ) ;
#3788=DIRECTION ( 'NONE',  ( -0.000000000000000000, -1.000000000000000000, -0.000000000000000000 ) ) ;
#3791=VECTOR ( 'NONE', #3047, 1000.000000000000114 ) ;
#3792=VECTOR ( 'NONE', #10358, 1000.000000000000000 ) ;
#3808=DIRECTION ( 'NONE',  ( 0.000000000000000000, 0.000000000000000000, 1.000000000000000000 ) ) ;
#3810=CARTESIAN_POINT ( 'NONE',  ( 12.21000000000000796, 0.000000000000000000, 0.2208617994340217328 ) ) ;
#3815=CYLINDRICAL_SURFACE ( 'NONE', #4205, 1.499999999999999556 ) ;
#3818=CARTESIAN_POINT ( 'NONE',  ( -8.222660081691577361, 3.000000000000000000, -8.549999999999998934 ) ) ;
#3820=AXIS2_PLACEMENT_3D ( 'NONE', #243, #8825, #3402 ) ;
#3824=ADVANCED_FACE ( 'NONE', ( #4356 ), #3383, .F. ) ;
#3827=CARTESIAN_POINT ( 'NONE',  ( 17.00000000000000355, 3.000000000000000000, -14.92471123914605435 ) ) ;
#3830=DIRECTION ( 'NONE',  ( -0.000000000000000000, -0.000000000000000000, 1.000000000000000000 ) ) ;
#3834=DIRECTION ( 'NONE',  ( -0.000000000000000000, -1.000000000000000000, -0.000000000000000000 ) ) ;
#3836=CARTESIAN_POINT ( 'NONE',  ( 20.00000000000000355, 0.000000000000000000, -14.92471123914604370 ) ) ;
#3838=ORIENTED_EDGE ( 'NONE', *, *, #607, .F. ) ;
#3852=FACE_OUTER_BOUND ( 'NONE', #6929, .T. ) ;
#3884=EDGE_LOOP ( 'NONE', ( #3470, #13020, #5382, #13016 ) ) ;
#3886=EDGE_LOOP ( 'NONE', ( #1834, #8435, #4979, #13296 ) ) ;
#3893=EDGE_CURVE ( 'NONE', #6080, #13469, #13207, .T. ) ;
#3901=CARTESIAN_POINT ( 'NONE',  ( 19.60942157306000766, 3.000000000000000000, 14.05941790610251374 ) ) ;
#3906=EDGE_CURVE ( 'NONE', #11282, #4803, #2154, .T. ) ;
#3909=EDGE_CURVE ( 'NONE', #5272, #2212, #12357, .T. ) ;
#3937=DIRECTION ( 'NONE',  ( 0.000000000000000000, 1.000000000000000000, 0.000000000000000000 ) ) ;
#3940=FACE_OUTER_BOUND ( 'NONE', #6664, .T. ) ;
#3946=DIRECTION ( 'NONE',  ( -1.000000000000000000, 0.000000000000000000, -0.000000000000000000 ) ) ;
#3955=CARTESIAN_POINT ( 'NONE',  ( 7.500000000000003553, 0.000000000000000000, 13.39999999999999858 ) ) ;
#3972=ORIENTED_EDGE ( 'NONE', *, *, #8368, .F. ) ;
#3974=EDGE_CURVE ( 'NONE', #1409, #732, #10896, .T. ) ;
#3999=AXIS2_PLACEMENT_3D ( 'NONE', #2382, #6578, #6517 ) ;
#4030=ORIENTED_EDGE ( 'NONE', *, *, #8822, .F. ) ;
#4033=VECTOR ( 'NONE', #526, 1000.000000000000000 ) ;
#4037=CARTESIAN_POINT ( 'NONE',  ( 7.500000000000003553, 0.000000000000000000, 4.899999999999997691 ) ) ;
#4044=AXIS2_PLACEMENT_3D ( 'NONE', #13404, #7212, #3062 ) ;
#4045=DIRECTION ( 'NONE',  ( 0.000000000000000000, 0.000000000000000000, -1.000000000000000000 ) ) ;
#4076=( GEOMETRIC_REPRESENTATION_CONTEXT ( 3 ) GLOBAL_UNCERTAINTY_ASSIGNED_CONTEXT ( ( #10811 ) ) GLOBAL_UNIT_ASSIGNED_CONTEXT ( ( #11858, #1390, #6555 ) ) REPRESENTATION_CONTEXT ( 'NONE', 'WORKASPACE' ) );
#4082=ADVANCED_FACE ( 'NONE', ( #1806 ), #6001, .F. ) ;
#4086=CARTESIAN_POINT ( 'NONE',  ( 6.000000000000008882, 3.000000000000000000, 25.50000000000000000 ) ) ;
#4112=ORIENTED_EDGE ( 'NONE', *, *, #10962, .F. ) ;
#4118=LINE ( 'NONE', #3219, #9468 ) ;
#4128=EDGE_CURVE ( 'NONE', #10071, #6484, #7575, .T. ) ;
#4139=VERTEX_POINT ( 'NONE', #8664 ) ;
#4163=CARTESIAN_POINT ( 'NONE',  ( 7.702138240596505092, 0.000000000000000000, -30.99999999999999289 ) ) ;
#4186=VECTOR ( 'NONE', #10479, 1000.000000000000000 ) ;
#4201=VERTEX_POINT ( 'NONE', #2137 ) ;
#4205=AXIS2_PLACEMENT_3D ( 'NONE', #1831, #10150, #7809 ) ;
#4206=EDGE_LOOP ( 'NONE', ( #9644, #8816, #4374, #8749, #8121, #13546, #10810, #5937, #4312, #12062, #6715, #4488, #12878, #7693, #11634, #12361 ) ) ;
#4208=DIRECTION ( 'NONE',  ( 1.000000000000000000, 0.000000000000000000, -1.269138026879196405E-16 ) ) ;
#4217=EDGE_LOOP ( 'NONE', ( #12111, #7925 ) ) ;
#4237=CIRCLE ( 'NONE', #3356, 3.000000000000002665 ) ;
#4253=EDGE_CURVE ( 'NONE', #9985, #11282, #8159, .T. ) ;
#4263=EDGE_LOOP ( 'NONE', ( #7861, #7877, #13073, #8192, #8962 ) ) ;
#4265=VECTOR ( 'NONE', #3834, 1000.000000000000000 ) ;
#4275=DIRECTION ( 'NONE',  ( -0.000000000000000000, -0.000000000000000000, 1.000000000000000000 ) ) ;
#4276=ORIENTED_EDGE ( 'NONE', *, *, #9463, .F. ) ;
#4280=VECTOR ( 'NONE', #1928, 1000.000000000000000 ) ;
#4295=ORIENTED_EDGE ( 'NONE', *, *, #11702, .T. ) ;
#4305=EDGE_CURVE ( 'NONE', #3370, #2212, #5846, .T. ) ;
#4312=ORIENTED_EDGE ( 'NONE', *, *, #2304, .F. ) ;
#4321=EDGE_CURVE ( 'NONE', #12313, #833, #1130, .T. ) ;
#4335=ORIENTED_EDGE ( 'NONE', *, *, #13266, .F. ) ;
#4355=CYLINDRICAL_SURFACE ( 'NONE', #11275, 1.500000000000001332 ) ;
#4356=FACE_OUTER_BOUND ( 'NONE', #3886, .T. ) ;
#4357=LINE ( 'NONE', #4420, #2002 ) ;
#4374=ORIENTED_EDGE ( 'NONE', *, *, #2060, .F. ) ;
#4380=CARTESIAN_POINT ( 'NONE',  ( -21.21140389626389222, 3.000000000000000000, 12.49772878833445056 ) ) ;
#4392=ORIENTED_EDGE ( 'NONE', *, *, #1631, .T. ) ;
#4393=FACE_OUTER_BOUND ( 'NONE', #147, .T. ) ;
#4399=FACE_OUTER_BOUND ( 'NONE', #4206, .T. ) ;
#4410=EDGE_CURVE ( 'NONE', #5397, #1515, #2005, .T. ) ;
#4420=CARTESIAN_POINT ( 'NONE',  ( 20.00000000000000355, 3.000000000000000000, -14.92471123914604370 ) ) ;
#4426=CIRCLE ( 'NONE', #9263, 2.999999999999999112 ) ;
#4429=ORIENTED_EDGE ( 'NONE', *, *, #7588, .F. ) ;
#4431=EDGE_LOOP ( 'NONE', ( #2661, #13080 ) ) ;
#4433=CARTESIAN_POINT ( 'NONE',  ( -10.88404822699983576, 3.000000000000000000, 29.60989680561421622 ) ) ;
#4434=LINE ( 'NONE', #6709, #13304 ) ;
#4448=CIRCLE ( 'NONE', #8397, 2.999999999999999112 ) ;
#4456=ORIENTED_EDGE ( 'NONE', *, *, #31, .T. ) ;
#4463=( GEOMETRIC_REPRESENTATION_CONTEXT ( 3 ) GLOBAL_UNCERTAINTY_ASSIGNED_CONTEXT ( ( #480 ) ) GLOBAL_UNIT_ASSIGNED_CONTEXT ( ( #13297, #8057, #1454 ) ) REPRESENTATION_CONTEXT ( 'NONE', 'WORKASPACE' ) );
#4474=AXIS2_PLACEMENT_3D ( 'NONE', #11456, #107, #5119 ) ;
#4480=CARTESIAN_POINT ( 'NONE',  ( -4.499999999999993783, 3.000000000000000000, 13.39999999999999858 ) ) ;
#4488=ORIENTED_EDGE ( 'NONE', *, *, #9258, .F. ) ;
#4494=CARTESIAN_POINT ( 'NONE',  ( -13.49999999999999645, 3.000000000000000000, -5.549999999999999822 ) ) ;
#4510=EDGE_CURVE ( 'NONE', #2370, #4741, #9419, .T. ) ;
#4516=AXIS2_PLACEMENT_3D ( 'NONE', #5042, #6909, #9242 ) ;
#4520=EDGE_LOOP ( 'NONE', ( #6322, #8328, #4429, #193 ) ) ;
#4555=FILL_AREA_STYLE_COLOUR ( '', #7803 ) ;
#4576=DIRECTION ( 'NONE',  ( 0.000000000000000000, 0.000000000000000000, 1.000000000000000000 ) ) ;
#4625=VERTEX_POINT ( 'NONE', #5218 ) ;
#4632=VERTEX_POINT ( 'NONE', #8446 ) ;
#4642=AXIS2_PLACEMENT_3D ( 'NONE', #6799, #5697, #5637 ) ;
#4644=FACE_OUTER_BOUND ( 'NONE', #5360, .T. ) ;
#4680=FACE_OUTER_BOUND ( 'NONE', #12737, .T. ) ;
#4681=DIRECTION ( 'NONE',  ( 0.000000000000000000, 1.000000000000000000, 0.000000000000000000 ) ) ;
#4697=DIRECTION ( 'NONE',  ( -0.000000000000000000, -1.000000000000000000, -0.000000000000000000 ) ) ;
#4701=AXIS2_PLACEMENT_3D ( 'NONE', #10365, #9260, #10441 ) ;
#4711=CARTESIAN_POINT ( 'NONE',  ( -21.21140389626389222, 3.000000000000000000, 12.49772878833445056 ) ) ;
#4713=CIRCLE ( 'NONE', #11534, 8.500000000000000000 ) ;
#4722=AXIS2_PLACEMENT_3D ( 'NONE', #1070, #48, #12850 ) ;
#4730=CARTESIAN_POINT ( 'NONE',  ( -5.250000000000000000, 3.000000000000000000, -29.44078293894052933 ) ) ;
#4731=EDGE_CURVE ( 'NONE', #4943, #10892, #247, .T. ) ;
#4734=AXIS2_PLACEMENT_3D ( 'NONE', #2914, #8280, #3808 ) ;
#4741=VERTEX_POINT ( 'NONE', #8774 ) ;
#4746=CARTESIAN_POINT ( 'NONE',  ( -13.49999999999999645, 3.000000000000000000, -7.049999999999998934 ) ) ;
#4752=CARTESIAN_POINT ( 'NONE',  ( -8.352599575481690408, 3.000000000000000000, 28.00000000000000000 ) ) ;
#4756=DIRECTION ( 'NONE',  ( -0.000000000000000000, -1.000000000000000000, -0.000000000000000000 ) ) ;
#4762=EDGE_CURVE ( 'NONE', #2558, #4834, #2454, .T. ) ;
#4803=VERTEX_POINT ( 'NONE', #8161 ) ;
#4813=CYLINDRICAL_SURFACE ( 'NONE', #2103, 12.00000000000000000 ) ;
#4815=PLANE ( 'NONE',  #12406 ) ;
#4825=CARTESIAN_POINT ( 'NONE',  ( -18.21140389626389577, 3.000000000000000000, -14.83930531255816376 ) ) ;
#4829=VECTOR ( 'NONE', #9766, 1000.000000000000000 ) ;
#4834=VERTEX_POINT ( 'NONE', #4037 ) ;
#4843=DIRECTION ( 'NONE',  ( 0.000000000000000000, 1.000000000000000000, 0.000000000000000000 ) ) ;
#4853=ORIENTED_EDGE ( 'NONE', *, *, #13161, .T. ) ;
#4855=DIRECTION ( 'NONE',  ( -0.000000000000000000, -1.000000000000000000, -0.000000000000000000 ) ) ;
#4862=LINE ( 'NONE', #13278, #2734 ) ;
#4869=ORIENTED_EDGE ( 'NONE', *, *, #936, .T. ) ;
#4873=AXIS2_PLACEMENT_3D ( 'NONE', #840, #1042, #13447 ) ;
#4882=VECTOR ( 'NONE', #11621, 1000.000000000000000 ) ;
#4883=ORIENTED_EDGE ( 'NONE', *, *, #3070, .T. ) ;
#4898=CIRCLE ( 'NONE', #2046, 2.000000000000000444 ) ;
#4904=CYLINDRICAL_SURFACE ( 'NONE', #1380, 5.486375544325371223 ) ;
#4912=EDGE_CURVE ( 'NONE', #1515, #1280, #7956, .T. ) ;
#4921=AXIS2_PLACEMENT_3D ( 'NONE', #2760, #6966, #11162 ) ;
#4930=EDGE_CURVE ( 'NONE', #9908, #748, #2417, .T. ) ;
#4943=VERTEX_POINT ( 'NONE', #2108 ) ;
#4978=ADVANCED_FACE ( 'NONE', ( #6367 ), #5210, .T. ) ;
#4979=ORIENTED_EDGE ( 'NONE', *, *, #2022, .F. ) ;
#4991=DIRECTION ( 'NONE',  ( 0.000000000000000000, 0.000000000000000000, -1.000000000000000000 ) ) ;
#4994=ORIENTED_EDGE ( 'NONE', *, *, #12268, .F. ) ;
#5002=CARTESIAN_POINT ( 'NONE',  ( 19.60942157306000766, 0.000000000000000000, 14.05941790610251374 ) ) ;
#5004=DIRECTION ( 'NONE',  ( -0.000000000000000000, -1.000000000000000000, -0.000000000000000000 ) ) ;
#5010=CYLINDRICAL_SURFACE ( 'NONE', #1811, 5.499999999999996447 ) ;
#5022=ORIENTED_EDGE ( 'NONE', *, *, #3909, .T. ) ;
#5027=VERTEX_POINT ( 'NONE', #3330 ) ;
#5028=CARTESIAN_POINT ( 'NONE',  ( -18.21140389626389577, 0.000000000000000000, -14.83930531255816376 ) ) ;
#5041=DIRECTION ( 'NONE',  ( -0.000000000000000000, -1.000000000000000000, -0.000000000000000000 ) ) ;
#5042=CARTESIAN_POINT ( 'NONE',  ( -8.222660081691577361, 3.000000000000000000, -5.549999999999999822 ) ) ;
#5051=LINE ( 'NONE', #11602, #11257 ) ;
#5054=ORIENTED_EDGE ( 'NONE', *, *, #6505, .T. ) ;
#5060=CARTESIAN_POINT ( 'NONE',  ( -13.28140389626389783, 3.000000000000000000, 13.39999999999999858 ) ) ;
#5061=PLANE ( 'NONE',  #10226 ) ;
#5063=ADVANCED_FACE ( 'NONE', ( #10772 ), #6572, .F. ) ;
#5066=DIRECTION ( 'NONE',  ( -0.000000000000000000, -1.000000000000000000, -0.000000000000000000 ) ) ;
#5069=EDGE_CURVE ( 'NONE', #45, #1742, #1318, .T. ) ;
#5075=CARTESIAN_POINT ( 'NONE',  ( 6.000000000000008882, 0.000000000000000000, 25.50000000000000000 ) ) ;
#5081=LINE ( 'NONE', #9278, #10552 ) ;
#5115=VECTOR ( 'NONE', #1199, 1000.000000000000000 ) ;
#5117=FACE_OUTER_BOUND ( 'NONE', #3391, .T. ) ;
#5119=DIRECTION ( 'NONE',  ( 0.000000000000000000, 0.000000000000000000, -1.000000000000000000 ) ) ;
#5145=ORIENTED_EDGE ( 'NONE', *, *, #10005, .F. ) ;
#5149=CYLINDRICAL_SURFACE ( 'NONE', #503, 3.000000000000002665 ) ;
#5156=DIRECTION ( 'NONE',  ( 0.000000000000000000, 0.000000000000000000, 1.000000000000000000 ) ) ;
#5175=CARTESIAN_POINT ( 'NONE',  ( 6.000000000000008882, 0.000000000000000000, 27.00000000000000000 ) ) ;
#5177=CARTESIAN_POINT ( 'NONE',  ( -5.250000000000000000, 3.000000000000000000, -27.94078293894052578 ) ) ;
#5178=LINE ( 'NONE', #10274, #8813 ) ;
#5192=CYLINDRICAL_SURFACE ( 'NONE', #3622, 8.500000000000000000 ) ;
#5194=DIRECTION ( 'NONE',  ( 0.000000000000000000, 0.000000000000000000, 1.000000000000000000 ) ) ;
#5203=DIRECTION ( 'NONE',  ( -0.000000000000000000, -1.000000000000000000, -0.000000000000000000 ) ) ;
#5210=CYLINDRICAL_SURFACE ( 'NONE', #13229, 2.999999999999999112 ) ;
#5218=CARTESIAN_POINT ( 'NONE',  ( 5.250000000000000000, 3.000000000000000000, -29.44078293894052933 ) ) ;
#5242=EDGE_CURVE ( 'NONE', #2397, #4803, #2428, .T. ) ;
#5250=DIRECTION ( 'NONE',  ( 0.000000000000000000, 0.000000000000000000, 1.000000000000000000 ) ) ;
#5251=DIRECTION ( 'NONE',  ( 0.000000000000000000, 0.000000000000000000, -1.000000000000000000 ) ) ;
#5254=DIRECTION ( 'NONE',  ( -0.000000000000000000, -1.000000000000000000, -0.000000000000000000 ) ) ;
#5256=VERTEX_POINT ( 'NONE', #6026 ) ;
#5259=VERTEX_POINT ( 'NONE', #10292 ) ;
#5272=VERTEX_POINT ( 'NONE', #11047 ) ;
#5277=VECTOR ( 'NONE', #1957, 1000.000000000000000 ) ;
#5280=SHAPE_DEFINITION_REPRESENTATION ( #3140, #11353 ) ;
#5291=DIRECTION ( 'NONE',  ( 0.000000000000000000, 1.000000000000000000, 0.000000000000000000 ) ) ;
#5294=FACE_BOUND ( 'NONE', #8165, .T. ) ;
#5300=DIRECTION ( 'NONE',  ( -0.000000000000000000, -1.000000000000000000, -0.000000000000000000 ) ) ;
#5301=CYLINDRICAL_SURFACE ( 'NONE', #1664, 2.999999999999999112 ) ;
#5303=ORIENTED_EDGE ( 'NONE', *, *, #6449, .T. ) ;
#5313=EDGE_CURVE ( 'NONE', #8988, #7608, #12114, .T. ) ;
#5314=CARTESIAN_POINT ( 'NONE',  ( 5.250000000000000000, 3.000000000000000000, -26.44078293894052578 ) ) ;
#5315=CARTESIAN_POINT ( 'NONE',  ( -5.250000000000000000, 3.000000000000000000, -26.44078293894052578 ) ) ;
#5319=DIRECTION ( 'NONE',  ( 0.000000000000000000, 0.000000000000000000, -1.000000000000000000 ) ) ;
#5331=AXIS2_PLACEMENT_3D ( 'NONE', #4752, #6878, #11086 ) ;
#5350=STYLED_ITEM('',(#13628),#8567);
#5351=CARTESIAN_POINT ( 'NONE',  ( -8.222660081691577361, 0.000000000000000000, -8.549999999999998934 ) ) ;
#5359=VERTEX_POINT ( 'NONE', #10743 ) ;
#5360=EDGE_LOOP ( 'NONE', ( #8753, #5663, #8991, #10419 ) ) ;
#5361=EDGE_LOOP ( 'NONE', ( #3409, #7730, #10004, #2463, #10754, #828, #6245, #8944, #13154, #7903, #308, #705, #13434, #2190, #10115, #13126 ) ) ;
#5366=VECTOR ( 'NONE', #11895, 1000.000000000000000 ) ;
#5368=AXIS2_PLACEMENT_3D ( 'NONE', #8965, #1410, #6908 ) ;
#5376=ORIENTED_EDGE ( 'NONE', *, *, #9364, .T. ) ;
#5382=ORIENTED_EDGE ( 'NONE', *, *, #12741, .T. ) ;
#5383=CARTESIAN_POINT ( 'NONE',  ( -8.352599575481674421, 3.000000000000000000, 31.00000000000000000 ) ) ;
#5384=DIRECTION ( 'NONE',  ( -0.000000000000000000, -1.000000000000000000, -0.000000000000000000 ) ) ;
#5385=DIRECTION ( 'NONE',  ( 0.000000000000000000, 0.000000000000000000, -1.000000000000000000 ) ) ;
#5397=VERTEX_POINT ( 'NONE', #11708 ) ;
#5424=ORIENTED_EDGE ( 'NONE', *, *, #2150, .F. ) ;
#5433=CARTESIAN_POINT ( 'NONE',  ( 13.50000000000000355, 0.000000000000000000, -7.050000000000000711 ) ) ;
#5436=DIRECTION ( 'NONE',  ( -0.000000000000000000, -1.000000000000000000, -0.000000000000000000 ) ) ;
#5443=ORIENTED_EDGE ( 'NONE', *, *, #12857, .F. ) ;
#5446=FACE_OUTER_BOUND ( 'NONE', #5971, .T. ) ;
#5447=CARTESIAN_POINT ( 'NONE',  ( -7.798201703419555209, 0.000000000000000000, -30.99999999999999289 ) ) ;
#5459=LINE ( 'NONE', #120, #13511 ) ;
#5483=ORIENTED_EDGE ( 'NONE', *, *, #2145, .F. ) ;
#5488=EDGE_CURVE ( 'NONE', #1714, #1838, #6841, .T. ) ;
#5491=FACE_OUTER_BOUND ( 'NONE', #6035, .T. ) ;
#5525=EDGE_LOOP ( 'NONE', ( #9368, #1166, #6307, #5902 ) ) ;
#5528=DIRECTION ( 'NONE',  ( -0.000000000000000000, -1.000000000000000000, -0.000000000000000000 ) ) ;
#5531=DIRECTION ( 'NONE',  ( 0.000000000000000000, 0.000000000000000000, 1.000000000000000000 ) ) ;
#5534=CYLINDRICAL_SURFACE ( 'NONE', #3123, 1.500000000000001332 ) ;
#5538=ORIENTED_EDGE ( 'NONE', *, *, #1122, .T. ) ;
#5539=CIRCLE ( 'NONE', #12386, 3.000000000000002665 ) ;
#5543=CARTESIAN_POINT ( 'NONE',  ( 6.000000000000008882, 0.000000000000000000, 28.50000000000000000 ) ) ;
#5545=CYLINDRICAL_SURFACE ( 'NONE', #12330, 5.486375544325371223 ) ;
#5559=EDGE_LOOP ( 'NONE', ( #10906, #7633, #8090, #12174 ) ) ;
#5561=DIRECTION ( 'NONE',  ( -0.000000000000000000, -1.000000000000000000, -0.000000000000000000 ) ) ;
#5573=CARTESIAN_POINT ( 'NONE',  ( 11.65525440103098731, 3.000000000000000000, 2.142386537870793362 ) ) ;
#5584=ORIENTED_EDGE ( 'NONE', *, *, #9428, .T. ) ;
#5599=VERTEX_POINT ( 'NONE', #12511 ) ;
#5602=AXIS2_PLACEMENT_3D ( 'NONE', #2309, #8426, #2168 ) ;
#5603=AXIS2_PLACEMENT_3D ( 'NONE', #6497, #1260, #371 ) ;
#5621=CARTESIAN_POINT ( 'NONE',  ( 8.208497377870827449, 0.000000000000000000, -8.550000000000002487 ) ) ;
#5632=ORIENTED_EDGE ( 'NONE', *, *, #4128, .F. ) ;
#5637=DIRECTION ( 'NONE',  ( 0.000000000000000000, 0.000000000000000000, 1.000000000000000000 ) ) ;
#5650=EDGE_CURVE ( 'NONE', #1736, #447, #2991, .T. ) ;
#5660=LINE ( 'NONE', #3319, #12823 ) ;
#5663=ORIENTED_EDGE ( 'NONE', *, *, #3906, .T. ) ;
#5697=DIRECTION ( 'NONE',  ( 0.000000000000000000, 1.000000000000000000, 0.000000000000000000 ) ) ;
#5699=CARTESIAN_POINT ( 'NONE',  ( 8.252687871541629860, 0.000000000000000000, 31.00000000000000000 ) ) ;
#5704=VERTEX_POINT ( 'NONE', #12637 ) ;
#5705=EDGE_CURVE ( 'NONE', #11639, #5259, #4357, .T. ) ;
#5712=DIRECTION ( 'NONE',  ( 1.000000000000000000, 0.000000000000000000, 0.000000000000000000 ) ) ;
#5729=EDGE_CURVE ( 'NONE', #4139, #4943, #452, .T. ) ;
#5741=DIRECTION ( 'NONE',  ( 0.000000000000000000, 0.000000000000000000, -1.000000000000000000 ) ) ;
#5773=DIRECTION ( 'NONE',  ( 0.000000000000000000, 0.000000000000000000, 1.000000000000000000 ) ) ;
#5774=DIRECTION ( 'NONE',  ( -1.000000000000000000, 0.000000000000000000, 1.261435711112880913E-16 ) ) ;
#5780=VECTOR ( 'NONE', #4756, 1000.000000000000000 ) ;
#5787=VECTOR ( 'NONE', #2932, 1000.000000000000000 ) ;
#5796=DIRECTION ( 'NONE',  ( 0.6204948238377419045, 0.000000000000000000, -0.7842105416216805791 ) ) ;
#5800=AXIS2_PLACEMENT_3D ( 'NONE', #3955, #7145, #11407 ) ;
#5801=VERTEX_POINT ( 'NONE', #7165 ) ;
#5814=VECTOR ( 'NONE', #554, 1000.000000000000000 ) ;
#5827=PLANE ( 'NONE',  #1859 ) ;
#5840=ORIENTED_EDGE ( 'NONE', *, *, #6745, .T. ) ;
#5846=LINE ( 'NONE', #1507, #12783 ) ;
#5868=CARTESIAN_POINT ( 'NONE',  ( -20.56403552112892896, 0.000000000000000000, -16.70078978407140013 ) ) ;
#5877=DIRECTION ( 'NONE',  ( 0.000000000000000000, 1.000000000000000000, -0.000000000000000000 ) ) ;
#5891=DIRECTION ( 'NONE',  ( 1.269138026879196405E-16, 0.000000000000000000, 1.000000000000000000 ) ) ;
#5902=ORIENTED_EDGE ( 'NONE', *, *, #4912, .T. ) ;
#5937=ORIENTED_EDGE ( 'NONE', *, *, #9942, .F. ) ;
#5950=FACE_OUTER_BOUND ( 'NONE', #2442, .T. ) ;
#5958=CARTESIAN_POINT ( 'NONE',  ( 8.252687871541629860, 3.000000000000000000, 31.00000000000000000 ) ) ;
#5971=EDGE_LOOP ( 'NONE', ( #577, #11400, #6411, #7253 ) ) ;
#5988=EDGE_CURVE ( 'NONE', #5397, #11577, #4118, .T. ) ;
#6001=CYLINDRICAL_SURFACE ( 'NONE', #3294, 1.500000000000001332 ) ;
#6014=EDGE_LOOP ( 'NONE', ( #5054, #12034, #9511, #4335 ) ) ;
#6026=CARTESIAN_POINT ( 'NONE',  ( -21.21140389626389577, 0.000000000000000000, -14.83930531255814955 ) ) ;
#6031=AXIS2_PLACEMENT_3D ( 'NONE', #5433, #3289, #7505 ) ;
#6035=EDGE_LOOP ( 'NONE', ( #9825, #4883, #5443, #4994 ) ) ;
#6065=ORIENTED_EDGE ( 'NONE', *, *, #1969, .T. ) ;
#6075=DIRECTION ( 'NONE',  ( -0.000000000000000000, -1.000000000000000000, -0.000000000000000000 ) ) ;
#6078=CARTESIAN_POINT ( 'NONE',  ( -13.28140389626389783, 3.000000000000000000, 13.39999999999999858 ) ) ;
#6080=VERTEX_POINT ( 'NONE', #9754 ) ;
#6085=ORIENTED_EDGE ( 'NONE', *, *, #4305, .F. ) ;
#6087=CARTESIAN_POINT ( 'NONE',  ( 13.50000000000000355, 3.000000000000000000, -8.550000000000000711 ) ) ;
#6089=FACE_OUTER_BOUND ( 'NONE', #3884, .T. ) ;
#6092=DIRECTION ( 'NONE',  ( -0.000000000000000000, -1.000000000000000000, -0.000000000000000000 ) ) ;
#6096=CARTESIAN_POINT ( 'NONE',  ( -5.250000000000000000, 3.000000000000000000, -29.44078293894052933 ) ) ;
#6173=LINE ( 'NONE', #3836, #6893 ) ;
#6175=EDGE_CURVE ( 'NONE', #180, #4632, #12182, .T. ) ;
#6187=VECTOR ( 'NONE', #8497, 1000.000000000000000 ) ;
#6194=ORIENTED_EDGE ( 'NONE', *, *, #6175, .T. ) ;
#6202=CARTESIAN_POINT ( 'NONE',  ( -8.352599575481674421, 0.000000000000000000, 31.00000000000000000 ) ) ;
#6205=CIRCLE ( 'NONE', #3122, 8.500000000000000000 ) ;
#6226=ORIENTED_EDGE ( 'NONE', *, *, #4321, .F. ) ;
#6228=ORIENTED_EDGE ( 'NONE', *, *, #1910, .F. ) ;
#6236=CARTESIAN_POINT ( 'NONE',  ( 10.14701493152832512, 3.000000000000000000, -29.73855628788322747 ) ) ;
#6243=FACE_OUTER_BOUND ( 'NONE', #4520, .T. ) ;
#6245=ORIENTED_EDGE ( 'NONE', *, *, #1115, .T. ) ;
#6255=AXIS2_PLACEMENT_3D ( 'NONE', #3417, #12870, #7629 ) ;
#6265=AXIS2_PLACEMENT_3D ( 'NONE', #9995, #4697, #704 ) ;
#6276=ORIENTED_EDGE ( 'NONE', *, *, #6505, .F. ) ;
#6286=DIRECTION ( 'NONE',  ( 0.000000000000000000, 0.000000000000000000, -1.000000000000000000 ) ) ;
#6288=FACE_OUTER_BOUND ( 'NONE', #8120, .T. ) ;
#6290=DIRECTION ( 'NONE',  ( 0.000000000000000000, 1.000000000000000000, 0.000000000000000000 ) ) ;
#6306=EDGE_CURVE ( 'NONE', #12681, #3357, #463, .T. ) ;
#6307=ORIENTED_EDGE ( 'NONE', *, *, #4410, .T. ) ;
#6309=DIRECTION ( 'NONE',  ( -0.000000000000000000, -1.000000000000000000, -0.000000000000000000 ) ) ;
#6313=LINE ( 'NONE', #10665, #1977 ) ;
#6321=LINE ( 'NONE', #265, #8642 ) ;
#6322=ORIENTED_EDGE ( 'NONE', *, *, #9888, .T. ) ;
#6338=LINE ( 'NONE', #280, #471 ) ;
#6355=EDGE_CURVE ( 'NONE', #11639, #2029, #4426, .T. ) ;
#6366=CARTESIAN_POINT ( 'NONE',  ( 10.86210944460165528, 3.000000000000000000, 29.48017534571043541 ) ) ;
#6367=FACE_OUTER_BOUND ( 'NONE', #3069, .T. ) ;
#6388=ORIENTED_EDGE ( 'NONE', *, *, #681, .T. ) ;
#6393=FACE_BOUND ( 'NONE', #7123, .T. ) ;
#6403=EDGE_LOOP ( 'NONE', ( #4295, #204, #10876, #12032 ) ) ;
#6411=ORIENTED_EDGE ( 'NONE', *, *, #4762, .T. ) ;
#6437=DIRECTION ( 'NONE',  ( -0.5366322685380731095, 0.000000000000000000, -0.8438162171727212613 ) ) ;
#6443=CARTESIAN_POINT ( 'NONE',  ( -13.49999999999999645, 3.000000000000000000, -5.549999999999999822 ) ) ;
#6449=EDGE_CURVE ( 'NONE', #12461, #2370, #7294, .T. ) ;
#6450=EDGE_CURVE ( 'NONE', #3357, #9908, #12717, .T. ) ;
#6470=AXIS2_PLACEMENT_3D ( 'NONE', #3552, #6940, #13069 ) ;
#6474=DIRECTION ( 'NONE',  ( 0.000000000000000000, 0.000000000000000000, 1.000000000000000000 ) ) ;
#6484=VERTEX_POINT ( 'NONE', #3260 ) ;
#6490=DIRECTION ( 'NONE',  ( 0.000000000000000000, 0.000000000000000000, -1.000000000000000000 ) ) ;
#6497=CARTESIAN_POINT ( 'NONE',  ( -5.250000000000000000, 0.000000000000000000, -27.94078293894052578 ) ) ;
#6505=EDGE_CURVE ( 'NONE', #7204, #7585, #1802, .T. ) ;
#6517=DIRECTION ( 'NONE',  ( 0.000000000000000000, 0.000000000000000000, -1.000000000000000000 ) ) ;
#6536=DIRECTION ( 'NONE',  ( 0.000000000000000000, -0.000000000000000000, -1.000000000000000000 ) ) ;
#6542=DIRECTION ( 'NONE',  ( 0.000000000000000000, 1.000000000000000000, 0.000000000000000000 ) ) ;
#6551=DIRECTION ( 'NONE',  ( 0.000000000000000000, 0.000000000000000000, 1.000000000000000000 ) ) ;
#6552=ORIENTED_EDGE ( 'NONE', *, *, #12415, .T. ) ;
#6555=( NAMED_UNIT ( * ) SI_UNIT ( $, .STERADIAN. ) SOLID_ANGLE_UNIT ( ) );
#6572=CYLINDRICAL_SURFACE ( 'NONE', #10334, 2.000000000000000444 ) ;
#6573=DIRECTION ( 'NONE',  ( 0.000000000000000000, 0.000000000000000000, 1.000000000000000000 ) ) ;
#6577=ORIENTED_EDGE ( 'NONE', *, *, #3335, .F. ) ;
#6578=DIRECTION ( 'NONE',  ( -0.000000000000000000, -1.000000000000000000, -0.000000000000000000 ) ) ;
#6588=EDGE_CURVE ( 'NONE', #2370, #12461, #7500, .T. ) ;
#6601=FACE_OUTER_BOUND ( 'NONE', #8316, .T. ) ;
#6603=CARTESIAN_POINT ( 'NONE',  ( 20.00000000000000355, 3.000000000000000000, -14.92471123914604370 ) ) ;
#6610=ORIENTED_EDGE ( 'NONE', *, *, #4510, .F. ) ;
#6612=ORIENTED_EDGE ( 'NONE', *, *, #9366, .T. ) ;
#6623=DIRECTION ( 'NONE',  ( -0.000000000000000000, -1.000000000000000000, -0.000000000000000000 ) ) ;
#6624=CARTESIAN_POINT ( 'NONE',  ( 6.000000000000008882, 3.000000000000000000, 27.00000000000000000 ) ) ;
#6645=VECTOR ( 'NONE', #10823, 1000.000000000000000 ) ;
#6663=ADVANCED_FACE ( 'NONE', ( #11048 ), #3815, .F. ) ;
#6664=EDGE_LOOP ( 'NONE', ( #9775, #9827, #13467, #6065 ) ) ;
#6665=ADVANCED_FACE ( 'NONE', ( #8018, #12238, #8088, #12164, #6845, #2712, #1549, #13184, #1622, #6992 ), #724, .F. ) ;
#6669=CYLINDRICAL_SURFACE ( 'NONE', #12404, 2.999999999999999112 ) ;
#6685=ORIENTED_EDGE ( 'NONE', *, *, #11824, .T. ) ;
#6687=ORIENTED_EDGE ( 'NONE', *, *, #3634, .F. ) ;
#6709=CARTESIAN_POINT ( 'NONE',  ( -13.49999999999999645, 3.000000000000000000, -8.549999999999998934 ) ) ;
#6715=ORIENTED_EDGE ( 'NONE', *, *, #2047, .F. ) ;
#6728=LINE ( 'NONE', #2800, #4265 ) ;
#6729=ORIENTED_EDGE ( 'NONE', *, *, #2283, .T. ) ;
#6738=DIRECTION ( 'NONE',  ( 0.000000000000000000, 0.000000000000000000, 1.000000000000000000 ) ) ;
#6745=EDGE_CURVE ( 'NONE', #10193, #930, #5051, .T. ) ;
#6754=CARTESIAN_POINT ( 'NONE',  ( 0.000000000000000000, 0.000000000000000000, 0.000000000000000000 ) ) ;
#6761=CARTESIAN_POINT ( 'NONE',  ( 7.500000000000004441, 0.000000000000000000, 21.89999999999999858 ) ) ;
#6764=ORIENTED_EDGE ( 'NONE', *, *, #10453, .T. ) ;
#6789=CARTESIAN_POINT ( 'NONE',  ( 3.469446951953614189E-15, 3.000000000000000000, -20.55000000000000071 ) ) ;
#6799=CARTESIAN_POINT ( 'NONE',  ( -5.250000000000000000, 3.000000000000000000, -27.94078293894052578 ) ) ;
#6802=CYLINDRICAL_SURFACE ( 'NONE', #5331, 2.999999999999992450 ) ;
#6803=LINE ( 'NONE', #3569, #3408 ) ;
#6807=EDGE_LOOP ( 'NONE', ( #98, #3243 ) ) ;
#6808=CIRCLE ( 'NONE', #13198, 2.999999999999999112 ) ;
#6813=EDGE_CURVE ( 'NONE', #9985, #2397, #12453, .T. ) ;
#6827=ORIENTED_EDGE ( 'NONE', *, *, #9593, .F. ) ;
#6830=EDGE_CURVE ( 'NONE', #2029, #10193, #7601, .T. ) ;
#6833=EDGE_LOOP ( 'NONE', ( #3156, #11885, #12792, #12383 ) ) ;
#6841=LINE ( 'NONE', #4711, #8785 ) ;
#6845=FACE_OUTER_BOUND ( 'NONE', #5361, .T. ) ;
#6859=CARTESIAN_POINT ( 'NONE',  ( -8.222660081691577361, 0.000000000000000000, -5.549999999999999822 ) ) ;
#6878=DIRECTION ( 'NONE',  ( -0.000000000000000000, -1.000000000000000000, -0.000000000000000000 ) ) ;
#6881=AXIS2_PLACEMENT_3D ( 'NONE', #1163, #5291, #10600 ) ;
#6885=EDGE_LOOP ( 'NONE', ( #7856, #6685 ) ) ;
#6893=VECTOR ( 'NONE', #10376, 1000.000000000000000 ) ;
#6897=LINE ( 'NONE', #5868, #9272 ) ;
#6908=DIRECTION ( 'NONE',  ( 0.000000000000000000, 0.000000000000000000, 1.000000000000000000 ) ) ;
#6909=DIRECTION ( 'NONE',  ( 1.055752450943286467E-16, -0.000000000000000000, 1.000000000000000000 ) ) ;
#6919=CARTESIAN_POINT ( 'NONE',  ( -7.798201703419567643, 3.000000000000000000, -27.99999999999999289 ) ) ;
#6924=ADVANCED_FACE ( 'NONE', ( #12963 ), #10562, .F. ) ;
#6929=EDGE_LOOP ( 'NONE', ( #10362, #7247, #12988, #8223 ) ) ;
#6940=DIRECTION ( 'NONE',  ( -0.000000000000000000, -1.000000000000000000, -0.000000000000000000 ) ) ;
#6946=CARTESIAN_POINT ( 'NONE',  ( 11.65525440103098731, 0.000000000000000000, 2.142386537870793362 ) ) ;
#6966=DIRECTION ( 'NONE',  ( -0.000000000000000000, -1.000000000000000000, -0.000000000000000000 ) ) ;
#6971=CARTESIAN_POINT ( 'NONE',  ( -7.798201703419555209, 3.000000000000000000, -30.99999999999999289 ) ) ;
#6992=FACE_BOUND ( 'NONE', #4263, .T. ) ;
#6993=CARTESIAN_POINT ( 'NONE',  ( 8.208497377870823897, 3.000000000000000000, -5.549999999999999822 ) ) ;
#7002=DIRECTION ( 'NONE',  ( -0.000000000000000000, -1.000000000000000000, -0.000000000000000000 ) ) ;
#7007=CARTESIAN_POINT ( 'NONE',  ( 5.250000000000000000, 3.000000000000000000, -27.94078293894052578 ) ) ;
#7008=CYLINDRICAL_SURFACE ( 'NONE', #6470, 13.50000000000000178 ) ;
#7021=DIRECTION ( 'NONE',  ( 0.000000000000000000, 1.000000000000000000, -0.000000000000000000 ) ) ;
#7040=CARTESIAN_POINT ( 'NONE',  ( -20.56403552112892896, 3.000000000000000000, -16.70078978407140013 ) ) ;
#7047=EDGE_CURVE ( 'NONE', #447, #4632, #6897, .T. ) ;
#7062=VECTOR ( 'NONE', #9524, 1000.000000000000000 ) ;
#7065=ORIENTED_EDGE ( 'NONE', *, *, #3974, .T. ) ;
#7066=EDGE_LOOP ( 'NONE', ( #12437, #3689, #3520, #5145 ) ) ;
#7072=DIRECTION ( 'NONE',  ( -0.000000000000000000, -1.000000000000000000, -0.000000000000000000 ) ) ;
#7079=ORIENTED_EDGE ( 'NONE', *, *, #7193, .F. ) ;
#7085=VECTOR ( 'NONE', #5203, 1000.000000000000000 ) ;
#7123=EDGE_LOOP ( 'NONE', ( #950, #9104 ) ) ;
#7136=EDGE_CURVE ( 'NONE', #3491, #2253, #9486, .T. ) ;
#7140=CIRCLE ( 'NONE', #1189, 1.500000000000001332 ) ;
#7145=DIRECTION ( 'NONE',  ( 0.000000000000000000, 1.000000000000000000, 0.000000000000000000 ) ) ;
#7146=VECTOR ( 'NONE', #1642, 1000.000000000000000 ) ;
#7149=LINE ( 'NONE', #7881, #2258 ) ;
#7157=DIRECTION ( 'NONE',  ( 0.000000000000000000, 0.000000000000000000, 1.000000000000000000 ) ) ;
#7165=CARTESIAN_POINT ( 'NONE',  ( 19.60942157306000766, 3.000000000000000000, 14.05941790610251374 ) ) ;
#7177=EDGE_CURVE ( 'NONE', #2682, #11250, #2008, .T. ) ;
#7182=EDGE_CURVE ( 'NONE', #8454, #2033, #3768, .T. ) ;
#7184=EDGE_CURVE ( 'NONE', #5027, #4139, #5178, .T. ) ;
#7186=DIRECTION ( 'NONE',  ( -0.000000000000000000, -1.000000000000000000, -0.000000000000000000 ) ) ;
#7189=EDGE_LOOP ( 'NONE', ( #12279, #9642, #2176, #13282 ) ) ;
#7193=EDGE_CURVE ( 'NONE', #5704, #10071, #11031, .T. ) ;
#7197=CYLINDRICAL_SURFACE ( 'NONE', #10336, 5.500000000000000000 ) ;
#7204=VERTEX_POINT ( 'NONE', #7578 ) ;
#7212=DIRECTION ( 'NONE',  ( 0.000000000000000000, 1.000000000000000000, 0.000000000000000000 ) ) ;
#7227=CARTESIAN_POINT ( 'NONE',  ( -12.38517345876401521, 3.000000000000000000, -12.42191571009144901 ) ) ;
#7247=ORIENTED_EDGE ( 'NONE', *, *, #3041, .T. ) ;
#7253=ORIENTED_EDGE ( 'NONE', *, *, #12986, .F. ) ;
#7255=FACE_OUTER_BOUND ( 'NONE', #3456, .T. ) ;
#7257=CARTESIAN_POINT ( 'NONE',  ( -10.88404822699983576, 3.000000000000000000, 29.60989680561421622 ) ) ;
#7284=DIRECTION ( 'NONE',  ( -0.000000000000000000, -1.000000000000000000, -0.000000000000000000 ) ) ;
#7294=CIRCLE ( 'NONE', #2445, 1.499999999999998668 ) ;
#7299=VERTEX_POINT ( 'NONE', #9773 ) ;
#7318=CIRCLE ( 'NONE', #6881, 1.499999999999998668 ) ;
#7335=CIRCLE ( 'NONE', #1613, 5.500000000000000000 ) ;
#7346=EDGE_CURVE ( 'NONE', #1668, #5256, #6338, .T. ) ;
#7362=CIRCLE ( 'NONE', #10879, 2.999999999999999112 ) ;
#7373=AXIS2_PLACEMENT_3D ( 'NONE', #3035, #11586, #8393 ) ;
#7376=CARTESIAN_POINT ( 'NONE',  ( 7.500000000000003553, 3.000000000000000000, 13.39999999999999858 ) ) ;
#7393=CARTESIAN_POINT ( 'NONE',  ( 7.500000000000003553, 3.000000000000000000, 13.39999999999999858 ) ) ;
#7437=ADVANCED_FACE ( 'NONE', ( #4680 ), #6802, .T. ) ;
#7451=EDGE_LOOP ( 'NONE', ( #7552, #2789, #8657, #932 ) ) ;
#7456=( NAMED_UNIT ( * ) PLANE_ANGLE_UNIT ( ) SI_UNIT ( $, .RADIAN. ) );
#7469=ORIENTED_EDGE ( 'NONE', *, *, #7896, .T. ) ;
#7500=CIRCLE ( 'NONE', #2660, 1.499999999999998668 ) ;
#7505=DIRECTION ( 'NONE',  ( 0.000000000000000000, 0.000000000000000000, 1.000000000000000000 ) ) ;
#7521=LINE ( 'NONE', #5314, #3131 ) ;
#7543=CARTESIAN_POINT ( 'NONE',  ( 7.702138240596516638, 3.000000000000000000, -27.99999999999999289 ) ) ;
#7547=VECTOR ( 'NONE', #3830, 1000.000000000000000 ) ;
#7552=ORIENTED_EDGE ( 'NONE', *, *, #7177, .T. ) ;
#7568=LINE ( 'NONE', #2464, #11283 ) ;
#7571=PLANE ( 'NONE',  #3082 ) ;
#7575=LINE ( 'NONE', #8524, #4186 ) ;
#7576=CARTESIAN_POINT ( 'NONE',  ( 17.00000000000000711, 3.000000000000000000, 12.57924256039205524 ) ) ;
#7578=CARTESIAN_POINT ( 'NONE',  ( -13.49999999999999645, 3.000000000000000000, -8.549999999999998934 ) ) ;
#7585=VERTEX_POINT ( 'NONE', #6443 ) ;
#7588=EDGE_CURVE ( 'NONE', #1714, #375, #5539, .T. ) ;
#7590=ORIENTED_EDGE ( 'NONE', *, *, #9416, .T. ) ;
#7596=CARTESIAN_POINT ( 'NONE',  ( 7.500000000000003553, 3.000000000000000000, 13.39999999999999858 ) ) ;
#7601=LINE ( 'NONE', #8612, #58 ) ;
#7606=VERTEX_POINT ( 'NONE', #8561 ) ;
#7608=VERTEX_POINT ( 'NONE', #9671 ) ;
#7615=DIRECTION ( 'NONE',  ( 0.000000000000000000, 1.000000000000000000, 0.000000000000000000 ) ) ;
#7624=CARTESIAN_POINT ( 'NONE',  ( -13.49999999999999645, 3.000000000000000000, -7.049999999999998934 ) ) ;
#7625=DIRECTION ( 'NONE',  ( 0.000000000000000000, 1.000000000000000000, 0.000000000000000000 ) ) ;
#7629=DIRECTION ( 'NONE',  ( 0.000000000000000000, 0.000000000000000000, -1.000000000000000000 ) ) ;
#7633=ORIENTED_EDGE ( 'NONE', *, *, #6745, .F. ) ;
#7638=VERTEX_POINT ( 'NONE', #11954 ) ;
#7642=DIRECTION ( 'NONE',  ( 0.000000000000000000, 0.000000000000000000, 1.000000000000000000 ) ) ;
#7674=DIRECTION ( 'NONE',  ( -0.000000000000000000, -1.000000000000000000, -0.000000000000000000 ) ) ;
#7689=DIRECTION ( 'NONE',  ( 0.000000000000000000, 0.000000000000000000, 1.000000000000000000 ) ) ;
#7693=ORIENTED_EDGE ( 'NONE', *, *, #11163, .F. ) ;
#7697=AXIS2_PLACEMENT_3D ( 'NONE', #7596, #1320, #8606 ) ;
#7700=ADVANCED_FACE ( 'NONE', ( #4644 ), #5534, .F. ) ;
#7717=AXIS2_PLACEMENT_3D ( 'NONE', #472, #10045, #6738 ) ;
#7719=PRESENTATION_STYLE_ASSIGNMENT (( #12005 ) ) ;
#7730=ORIENTED_EDGE ( 'NONE', *, *, #12949, .T. ) ;
#7739=ORIENTED_EDGE ( 'NONE', *, *, #9942, .T. ) ;
#7756=AXIS2_PLACEMENT_3D ( 'NONE', #9456, #8348, #13468 ) ;
#7759=CARTESIAN_POINT ( 'NONE',  ( -8.352599575481674421, 3.000000000000000000, 31.00000000000000000 ) ) ;
#7782=ORIENTED_EDGE ( 'NONE', *, *, #2472, .F. ) ;
#7803=COLOUR_RGB ( '',0.7803921568627451011, 0.7607843137254901578, 0.7411764705882353255 ) ;
#7809=DIRECTION ( 'NONE',  ( 0.000000000000000000, 0.000000000000000000, -1.000000000000000000 ) ) ;
#7820=CARTESIAN_POINT ( 'NONE',  ( 3.469446951953614189E-15, 3.000000000000000000, -7.049999999999999822 ) ) ;
#7825=ADVANCED_FACE ( 'NONE', ( #8149 ), #726, .F. ) ;
#7849=EDGE_LOOP ( 'NONE', ( #469, #11633, #7782, #8220 ) ) ;
#7856=ORIENTED_EDGE ( 'NONE', *, *, #5242, .T. ) ;
#7861=ORIENTED_EDGE ( 'NONE', *, *, #4731, .F. ) ;
#7874=CARTESIAN_POINT ( 'NONE',  ( -13.28140389626389783, 3.000000000000000000, -1.567980996311402420 ) ) ;
#7877=ORIENTED_EDGE ( 'NONE', *, *, #5729, .F. ) ;
#7881=CARTESIAN_POINT ( 'NONE',  ( -5.999999999999991118, 3.000000000000000000, 25.50000000000000000 ) ) ;
#7887=ORIENTED_EDGE ( 'NONE', *, *, #4410, .F. ) ;
#7896=EDGE_CURVE ( 'NONE', #5259, #10212, #1600, .T. ) ;
#7903=ORIENTED_EDGE ( 'NONE', *, *, #607, .T. ) ;
#7911=EDGE_CURVE ( 'NONE', #7608, #3702, #11401, .T. ) ;
#7919=AXIS2_PLACEMENT_3D ( 'NONE', #6624, #10824, #2218 ) ;
#7925=ORIENTED_EDGE ( 'NONE', *, *, #11133, .F. ) ;
#7929=AXIS2_PLACEMENT_3D ( 'NONE', #1257, #231, #5773 ) ;
#7943=CARTESIAN_POINT ( 'NONE',  ( -5.999999999999991118, 3.000000000000000000, 27.00000000000000000 ) ) ;
#7951=EDGE_LOOP ( 'NONE', ( #9131, #9027, #5584, #10831 ) ) ;
#7956=LINE ( 'NONE', #11136, #12552 ) ;
#7963=CARTESIAN_POINT ( 'NONE',  ( -8.222660081691577361, 3.000000000000000000, -5.549999999999999822 ) ) ;
#7967=EDGE_LOOP ( 'NONE', ( #9008, #8423, #10018, #10998 ) ) ;
#7971=AXIS2_PLACEMENT_3D ( 'NONE', #2153, #3108, #5250 ) ;
#7982=CARTESIAN_POINT ( 'NONE',  ( 19.60942157306000766, 3.000000000000000000, 14.05941790610251374 ) ) ;
#7984=ORIENTED_EDGE ( 'NONE', *, *, #5488, .F. ) ;
#7989=DIRECTION ( 'NONE',  ( -0.000000000000000000, -1.000000000000000000, -0.000000000000000000 ) ) ;
#8018=FACE_BOUND ( 'NONE', #12439, .T. ) ;
#8021=EDGE_CURVE ( 'NONE', #10212, #930, #3518, .T. ) ;
#8027=EDGE_CURVE ( 'NONE', #4625, #10097, #5660, .T. ) ;
#8029=DIRECTION ( 'NONE',  ( 0.000000000000000000, 0.000000000000000000, -1.000000000000000000 ) ) ;
#8037=LINE ( 'NONE', #7963, #7146 ) ;
#8052=DIRECTION ( 'NONE',  ( 0.000000000000000000, 0.000000000000000000, 1.000000000000000000 ) ) ;
#8057=( NAMED_UNIT ( * ) PLANE_ANGLE_UNIT ( ) SI_UNIT ( $, .RADIAN. ) );
#8075=VERTEX_POINT ( 'NONE', #176 ) ;
#8088=FACE_BOUND ( 'NONE', #3422, .T. ) ;
#8090=ORIENTED_EDGE ( 'NONE', *, *, #6830, .F. ) ;
#8100=CARTESIAN_POINT ( 'NONE',  ( -13.49999999999999645, 0.000000000000000000, -7.049999999999998934 ) ) ;
#8104=AXIS2_PLACEMENT_3D ( 'NONE', #5028, #834, #8127 ) ;
#8113=CARTESIAN_POINT ( 'NONE',  ( -13.49999999999999645, 3.000000000000000000, -7.049999999999998934 ) ) ;
#8120=EDGE_LOOP ( 'NONE', ( #2517, #1934, #3763, #6610 ) ) ;
#8121=ORIENTED_EDGE ( 'NONE', *, *, #7896, .F. ) ;
#8122=CARTESIAN_POINT ( 'NONE',  ( 12.37962962962963864, 0.000000000000000000, -12.43467921358330663 ) ) ;
#8127=DIRECTION ( 'NONE',  ( 0.000000000000000000, 0.000000000000000000, -1.000000000000000000 ) ) ;
#8133=FACE_OUTER_BOUND ( 'NONE', #6833, .T. ) ;
#8140=AXIS2_PLACEMENT_3D ( 'NONE', #7943, #10683, #9639 ) ;
#8143=PLANE ( 'NONE',  #2420 ) ;
#8145=CARTESIAN_POINT ( 'NONE',  ( 3.469446951953614189E-15, 0.000000000000000000, -7.049999999999999822 ) ) ;
#8149=FACE_OUTER_BOUND ( 'NONE', #12776, .T. ) ;
#8158=LINE ( 'NONE', #5060, #5787 ) ;
#8159=CIRCLE ( 'NONE', #4642, 1.500000000000001332 ) ;
#8161=CARTESIAN_POINT ( 'NONE',  ( -5.250000000000000000, 0.000000000000000000, -26.44078293894052578 ) ) ;
#8165=EDGE_LOOP ( 'NONE', ( #13450, #11071, #6764, #877, #8402 ) ) ;
#8183=ADVANCED_FACE ( 'NONE', ( #1678 ), #4904, .T. ) ;
#8189=CIRCLE ( 'NONE', #7971, 5.500000000000000000 ) ;
#8192=ORIENTED_EDGE ( 'NONE', *, *, #9428, .F. ) ;
#8213=LINE ( 'NONE', #2989, #3791 ) ;
#8220=ORIENTED_EDGE ( 'NONE', *, *, #4305, .T. ) ;
#8222=VECTOR ( 'NONE', #12962, 1000.000000000000000 ) ;
#8223=ORIENTED_EDGE ( 'NONE', *, *, #1631, .F. ) ;
#8230=FACE_OUTER_BOUND ( 'NONE', #5559, .T. ) ;
#8240=VERTEX_POINT ( 'NONE', #6761 ) ;
#8241=LINE ( 'NONE', #3901, #7085 ) ;
#8253=LINE ( 'NONE', #7227, #4280 ) ;
#8262=EDGE_LOOP ( 'NONE', ( #7739, #12425, #3838, #11921 ) ) ;
#8269=DIRECTION ( 'NONE',  ( 0.000000000000000000, 1.000000000000000000, 0.000000000000000000 ) ) ;
#8275=ORIENTED_EDGE ( 'NONE', *, *, #12334, .T. ) ;
#8280=DIRECTION ( 'NONE',  ( 0.000000000000000000, 1.000000000000000000, 0.000000000000000000 ) ) ;
#8316=EDGE_LOOP ( 'NONE', ( #8486, #4869, #12720, #10886 ) ) ;
#8323=DIRECTION ( 'NONE',  ( 0.000000000000000000, 1.000000000000000000, 0.000000000000000000 ) ) ;
#8328=ORIENTED_EDGE ( 'NONE', *, *, #2363, .F. ) ;
#8333=CARTESIAN_POINT ( 'NONE',  ( -10.15083332828461771, 0.000000000000000000, -29.86148447151320795 ) ) ;
#8348=DIRECTION ( 'NONE',  ( 0.000000000000000000, 1.000000000000000000, -0.000000000000000000 ) ) ;
#8365=VERTEX_POINT ( 'NONE', #6078 ) ;
#8368=EDGE_CURVE ( 'NONE', #833, #1513, #7335, .T. ) ;
#8372=CYLINDRICAL_SURFACE ( 'NONE', #962, 1.500000000000001332 ) ;
#8393=DIRECTION ( 'NONE',  ( 0.000000000000000000, 0.000000000000000000, 1.000000000000000000 ) ) ;
#8397=AXIS2_PLACEMENT_3D ( 'NONE', #4825, #2492, #13311 ) ;
#8399=ORIENTED_EDGE ( 'NONE', *, *, #3385, .F. ) ;
#8402=ORIENTED_EDGE ( 'NONE', *, *, #6450, .T. ) ;
#8423=ORIENTED_EDGE ( 'NONE', *, *, #1969, .F. ) ;
#8426=DIRECTION ( 'NONE',  ( 0.000000000000000000, 1.000000000000000000, 0.000000000000000000 ) ) ;
#8435=ORIENTED_EDGE ( 'NONE', *, *, #13185, .T. ) ;
#8446=CARTESIAN_POINT ( 'NONE',  ( -20.56403552112892896, 0.000000000000000000, -16.70078978407140013 ) ) ;
#8454=VERTEX_POINT ( 'NONE', #4480 ) ;
#8460=FACE_BOUND ( 'NONE', #13581, .T. ) ;
#8480=DIRECTION ( 'NONE',  ( 0.000000000000000000, 0.000000000000000000, -1.000000000000000000 ) ) ;
#8486=ORIENTED_EDGE ( 'NONE', *, *, #10686, .F. ) ;
#8496=DIRECTION ( 'NONE',  ( -0.000000000000000000, -1.000000000000000000, -0.000000000000000000 ) ) ;
#8497=DIRECTION ( 'NONE',  ( 1.000000000000000000, 0.000000000000000000, 0.000000000000000000 ) ) ;
#8507=LINE ( 'NONE', #1081, #11431 ) ;
#8524=CARTESIAN_POINT ( 'NONE',  ( 10.86210944460165528, 3.000000000000000000, 29.48017534571043541 ) ) ;
#8537=EDGE_CURVE ( 'NONE', #1515, #8365, #9507, .T. ) ;
#8555=DIRECTION ( 'NONE',  ( -0.000000000000000000, -1.000000000000000000, -0.000000000000000000 ) ) ;
#8561=CARTESIAN_POINT ( 'NONE',  ( 7.702138240596505092, 3.000000000000000000, -30.99999999999999289 ) ) ;
#8564=EDGE_CURVE ( 'NONE', #2964, #2682, #2815, .T. ) ;
#8566=CARTESIAN_POINT ( 'NONE',  ( 3.469446951953614189E-15, 0.000000000000000000, -7.049999999999999822 ) ) ;
#8567=MANIFOLD_SOLID_BREP ( 'Base-Flange1', #13019 ) ;
#8593=ADVANCED_FACE ( 'NONE', ( #3572 ), #4815, .F. ) ;
#8602=ORIENTED_EDGE ( 'NONE', *, *, #2060, .T. ) ;
#8606=DIRECTION ( 'NONE',  ( 0.000000000000000000, 0.000000000000000000, -1.000000000000000000 ) ) ;
#8612=CARTESIAN_POINT ( 'NONE',  ( 10.14701493152832512, 3.000000000000000000, -29.73855628788322747 ) ) ;
#8624=CARTESIAN_POINT ( 'NONE',  ( 5.250000000000000000, 0.000000000000000000, -27.94078293894052578 ) ) ;
#8630=CIRCLE ( 'NONE', #13271, 2.999999999999992450 ) ;
#8642=VECTOR ( 'NONE', #1087, 1000.000000000000000 ) ;
#8657=ORIENTED_EDGE ( 'NONE', *, *, #11594, .F. ) ;
#8664=CARTESIAN_POINT ( 'NONE',  ( 8.208497377870827449, 3.000000000000000000, -8.550000000000002487 ) ) ;
#8667=CARTESIAN_POINT ( 'NONE',  ( -4.499999999999993783, 3.000000000000000000, 13.39999999999999858 ) ) ;
#8672=CIRCLE ( 'NONE', #2744, 5.486375544325371223 ) ;
#8674=AXIS2_PLACEMENT_3D ( 'NONE', #7007, #6290, #13277 ) ;
#8676=AXIS2_PLACEMENT_3D ( 'NONE', #11251, #3937, #11450 ) ;
#8679=ORIENTED_EDGE ( 'NONE', *, *, #92, .F. ) ;
#8686=AXIS2_PLACEMENT_3D ( 'NONE', #12674, #12732, #7689 ) ;
#8688=DIRECTION ( 'NONE',  ( -0.5795187626277481518, -0.000000000000000000, -0.8149588969772669778 ) ) ;
#8693=ORIENTED_EDGE ( 'NONE', *, *, #3893, .T. ) ;
#8697=DIRECTION ( 'NONE',  ( 0.000000000000000000, 1.000000000000000000, 0.000000000000000000 ) ) ;
#8703=DIRECTION ( 'NONE',  ( -0.000000000000000000, -1.000000000000000000, -0.000000000000000000 ) ) ;
#8705=ORIENTED_EDGE ( 'NONE', *, *, #7346, .T. ) ;
#8707=DIRECTION ( 'NONE',  ( 0.000000000000000000, 0.000000000000000000, 1.000000000000000000 ) ) ;
#8723=DIRECTION ( 'NONE',  ( -0.000000000000000000, -1.000000000000000000, -0.000000000000000000 ) ) ;
#8726=CARTESIAN_POINT ( 'NONE',  ( 7.500000000000003553, 3.000000000000000000, 1.399999999999998579 ) ) ;
#8746=LINE ( 'NONE', #4494, #8222 ) ;
#8749=ORIENTED_EDGE ( 'NONE', *, *, #8021, .F. ) ;
#8753=ORIENTED_EDGE ( 'NONE', *, *, #4253, .T. ) ;
#8760=DIRECTION ( 'NONE',  ( 0.000000000000000000, 0.000000000000000000, 1.000000000000000000 ) ) ;
#8770=VERTEX_POINT ( 'NONE', #10790 ) ;
#8774=CARTESIAN_POINT ( 'NONE',  ( 13.50000000000000355, 0.000000000000000000, -8.550000000000000711 ) ) ;
#8785=VECTOR ( 'NONE', #1479, 1000.000000000000000 ) ;
#8813=VECTOR ( 'NONE', #9381, 1000.000000000000000 ) ;
#8816=ORIENTED_EDGE ( 'NONE', *, *, #9416, .F. ) ;
#8822=EDGE_CURVE ( 'NONE', #7606, #1409, #6321, .T. ) ;
#8825=DIRECTION ( 'NONE',  ( 0.000000000000000000, 1.000000000000000000, 0.000000000000000000 ) ) ;
#8854=VECTOR ( 'NONE', #5891, 1000.000000000000000 ) ;
#8858=MECHANICAL_DESIGN_GEOMETRIC_PRESENTATION_REPRESENTATION('',(#5350),#4463);
#8864=AXIS2_PLACEMENT_3D ( 'NONE', #8624, #8697, #3462 ) ;
#8877=AXIS2_PLACEMENT_3D ( 'NONE', #9201, #2940, #13352 ) ;
#8884=APPLICATION_CONTEXT ( 'automotive_design' ) ;
#8907=DIRECTION ( 'NONE',  ( 0.000000000000000000, 1.000000000000000000, 0.000000000000000000 ) ) ;
#8933=DIRECTION ( 'NONE',  ( 0.000000000000000000, 0.000000000000000000, -1.000000000000000000 ) ) ;
#8942=DIRECTION ( 'NONE',  ( -0.8698071910200015910, 0.000000000000000000, -0.4933917819034833729 ) ) ;
#8944=ORIENTED_EDGE ( 'NONE', *, *, #11594, .T. ) ;
#8947=ORIENTED_EDGE ( 'NONE', *, *, #10913, .F. ) ;
#8948=EDGE_CURVE ( 'NONE', #10892, #10888, #3686, .T. ) ;
#8962=ORIENTED_EDGE ( 'NONE', *, *, #2283, .F. ) ;
#8965=CARTESIAN_POINT ( 'NONE',  ( 3.469446951953614189E-15, 3.000000000000000000, -7.049999999999999822 ) ) ;
#8973=DIRECTION ( 'NONE',  ( -0.000000000000000000, -1.000000000000000000, -0.000000000000000000 ) ) ;
#8988=VERTEX_POINT ( 'NONE', #11352 ) ;
#8991=ORIENTED_EDGE ( 'NONE', *, *, #5242, .F. ) ;
#8992=CIRCLE ( 'NONE', #9875, 12.00000000000000000 ) ;
#9001=CARTESIAN_POINT ( 'NONE',  ( 7.500000000000003553, 3.000000000000000000, 13.39999999999999858 ) ) ;
#9003=DIRECTION ( 'NONE',  ( -0.4933917819034833174, 0.000000000000000000, 0.8698071910200014800 ) ) ;
#9008=ORIENTED_EDGE ( 'NONE', *, *, #13161, .F. ) ;
#9027=ORIENTED_EDGE ( 'NONE', *, *, #11300, .F. ) ;
#9034=EDGE_CURVE ( 'NONE', #2212, #5259, #6173, .T. ) ;
#9054=LINE ( 'NONE', #13272, #7547 ) ;
#9069=DIRECTION ( 'NONE',  ( -0.000000000000000000, -1.000000000000000000, -0.000000000000000000 ) ) ;
#9087=EDGE_CURVE ( 'NONE', #1251, #7638, #4898, .T. ) ;
#9104=ORIENTED_EDGE ( 'NONE', *, *, #12088, .T. ) ;
#9121=CARTESIAN_POINT ( 'NONE',  ( 13.50000000000000355, 3.000000000000000000, -7.050000000000000711 ) ) ;
#9131=ORIENTED_EDGE ( 'NONE', *, *, #6306, .F. ) ;
#9138=CIRCLE ( 'NONE', #8686, 4.390701948131951582 ) ;
#9174=CARTESIAN_POINT ( 'NONE',  ( -20.74285254778206067, 3.000000000000000000, 14.10762559394868099 ) ) ;
#9201=CARTESIAN_POINT ( 'NONE',  ( 7.500000000000003553, 0.000000000000000000, 13.39999999999999858 ) ) ;
#9218=ORIENTED_EDGE ( 'NONE', *, *, #1829, .T. ) ;
#9242=DIRECTION ( 'NONE',  ( 1.000000000000000000, 0.000000000000000000, -1.055752450943286467E-16 ) ) ;
#9258=EDGE_CURVE ( 'NONE', #2349, #5599, #8213, .T. ) ;
#9260=DIRECTION ( 'NONE',  ( 0.000000000000000000, 1.000000000000000000, 0.000000000000000000 ) ) ;
#9262=CARTESIAN_POINT ( 'NONE',  ( 10.14701493152832512, 3.000000000000000000, -29.73855628788322747 ) ) ;
#9263=AXIS2_PLACEMENT_3D ( 'NONE', #3206, #3067, #3009 ) ;
#9265=FACE_OUTER_BOUND ( 'NONE', #9290, .T. ) ;
#9272=VECTOR ( 'NONE', #10900, 1000.000000000000227 ) ;
#9278=CARTESIAN_POINT ( 'NONE',  ( -8.222660081691577361, 3.000000000000000000, -8.549999999999998934 ) ) ;
#9290=EDGE_LOOP ( 'NONE', ( #2835, #5424, #135, #2000 ) ) ;
#9315=AXIS2_PLACEMENT_3D ( 'NONE', #1694, #802, #4991 ) ;
#9329=CIRCLE ( 'NONE', #5800, 8.500000000000000000 ) ;
#9331=CARTESIAN_POINT ( 'NONE',  ( -5.999999999999991118, 3.000000000000000000, 28.50000000000000000 ) ) ;
#9332=CIRCLE ( 'NONE', #3378, 2.999999999999999112 ) ;
#9333=ORIENTED_EDGE ( 'NONE', *, *, #11824, .F. ) ;
#9360=VECTOR ( 'NONE', #5436, 1000.000000000000000 ) ;
#9364=EDGE_CURVE ( 'NONE', #4139, #9908, #991, .T. ) ;
#9366=EDGE_CURVE ( 'NONE', #7638, #12626, #8189, .T. ) ;
#9368=ORIENTED_EDGE ( 'NONE', *, *, #13274, .F. ) ;
#9380=ADVANCED_FACE ( 'NONE', ( #12761 ), #10696, .F. ) ;
#9381=DIRECTION ( 'NONE',  ( 1.000000000000000000, 0.000000000000000000, 0.000000000000000000 ) ) ;
#9396=ADVANCED_FACE ( 'NONE', ( #3382 ), #4355, .F. ) ;
#9409=DIRECTION ( 'NONE',  ( -0.000000000000000000, -1.000000000000000000, -0.000000000000000000 ) ) ;
#9416=EDGE_CURVE ( 'NONE', #13159, #732, #2358, .T. ) ;
#9419=LINE ( 'NONE', #12537, #12367 ) ;
#9428=EDGE_CURVE ( 'NONE', #10734, #5027, #716, .T. ) ;
#9456=CARTESIAN_POINT ( 'NONE',  ( 17.00000000000000355, 0.000000000000000000, -14.92471123914605435 ) ) ;
#9463=EDGE_CURVE ( 'NONE', #3023, #12683, #7521, .T. ) ;
#9466=CARTESIAN_POINT ( 'NONE',  ( 7.500000000000004441, 3.000000000000000000, 21.89999999999999858 ) ) ;
#9468=VECTOR ( 'NONE', #1989, 1000.000000000000000 ) ;
#9474=ORIENTED_EDGE ( 'NONE', *, *, #2145, .T. ) ;
#9486=CIRCLE ( 'NONE', #9924, 1.499999999999998668 ) ;
#9495=CIRCLE ( 'NONE', #12153, 13.50000000000000178 ) ;
#9506=CIRCLE ( 'NONE', #3560, 1.499999999999998668 ) ;
#9507=LINE ( 'NONE', #11850, #10411 ) ;
#9511=ORIENTED_EDGE ( 'NONE', *, *, #681, .F. ) ;
#9513=EDGE_CURVE ( 'NONE', #12626, #11577, #13166, .T. ) ;
#9521=VECTOR ( 'NONE', #11135, 1000.000000000000000 ) ;
#9524=DIRECTION ( 'NONE',  ( -0.000000000000000000, -1.000000000000000000, -0.000000000000000000 ) ) ;
#9534=CIRCLE ( 'NONE', #4921, 12.00000000000000000 ) ;
#9556=AXIS2_PLACEMENT_3D ( 'NONE', #583, #5877, #1614 ) ;
#9572=EDGE_LOOP ( 'NONE', ( #477, #1005, #485, #9333 ) ) ;
#9588=CARTESIAN_POINT ( 'NONE',  ( 20.00000000000000355, 3.000000000000000000, -14.92471123914604370 ) ) ;
#9591=CARTESIAN_POINT ( 'NONE',  ( -13.49999999999999645, 3.000000000000000000, -7.049999999999998934 ) ) ;
#9592=DIRECTION ( 'NONE',  ( 1.000000000000000000, -0.000000000000000000, 0.000000000000000000 ) ) ;
#9593=EDGE_CURVE ( 'NONE', #180, #1668, #4448, .T. ) ;
#9599=DIRECTION ( 'NONE',  ( -0.000000000000000000, -1.000000000000000000, -0.000000000000000000 ) ) ;
#9612=CARTESIAN_POINT ( 'NONE',  ( -5.250000000000000000, 3.000000000000000000, -27.94078293894052578 ) ) ;
#9639=DIRECTION ( 'NONE',  ( 0.000000000000000000, 0.000000000000000000, 1.000000000000000000 ) ) ;
#9642=ORIENTED_EDGE ( 'NONE', *, *, #11133, .T. ) ;
#9644=ORIENTED_EDGE ( 'NONE', *, *, #11479, .F. ) ;
#9661=ORIENTED_EDGE ( 'NONE', *, *, #2381, .T. ) ;
#9668=DIRECTION ( 'NONE',  ( 0.000000000000000000, 1.000000000000000000, 0.000000000000000000 ) ) ;
#9671=CARTESIAN_POINT ( 'NONE',  ( -5.999999999999991118, 3.000000000000000000, 28.50000000000000000 ) ) ;
#9672=VECTOR ( 'NONE', #5066, 1000.000000000000000 ) ;
#9686=CARTESIAN_POINT ( 'NONE',  ( 5.250000000000000000, 0.000000000000000000, -26.44078293894052578 ) ) ;
#9699=CYLINDRICAL_SURFACE ( 'NONE', #2623, 12.00000000000000000 ) ;
#9701=CARTESIAN_POINT ( 'NONE',  ( 6.000000000000008882, 3.000000000000000000, 27.00000000000000000 ) ) ;
#9716=SURFACE_STYLE_FILL_AREA ( #2489 ) ;
#9728=EDGE_LOOP ( 'NONE', ( #2294, #6729, #10216, #2371 ) ) ;
#9731=AXIS2_PLACEMENT_3D ( 'NONE', #11859, #104, #8480 ) ;
#9747=AXIS2_PLACEMENT_3D ( 'NONE', #3818, #10083, #3946 ) ;
#9752=DIRECTION ( 'NONE',  ( 0.000000000000000000, 0.000000000000000000, 1.000000000000000000 ) ) ;
#9754=CARTESIAN_POINT ( 'NONE',  ( 6.000000000000008882, 3.000000000000000000, 28.50000000000000000 ) ) ;
#9766=DIRECTION ( 'NONE',  ( -0.000000000000000000, -1.000000000000000000, -0.000000000000000000 ) ) ;
#9773=CARTESIAN_POINT ( 'NONE',  ( -4.499999999999993783, 0.000000000000000000, 13.39999999999999858 ) ) ;
#9775=ORIENTED_EDGE ( 'NONE', *, *, #10040, .F. ) ;
#9776=EDGE_CURVE ( 'NONE', #1742, #45, #12405, .T. ) ;
#9813=EDGE_LOOP ( 'NONE', ( #2515, #77 ) ) ;
#9816=ORIENTED_EDGE ( 'NONE', *, *, #12822, .F. ) ;
#9825=ORIENTED_EDGE ( 'NONE', *, *, #7182, .T. ) ;
#9827=ORIENTED_EDGE ( 'NONE', *, *, #4912, .F. ) ;
#9842=DIRECTION ( 'NONE',  ( 0.000000000000000000, 1.000000000000000000, 0.000000000000000000 ) ) ;
#9870=CARTESIAN_POINT ( 'NONE',  ( 13.50000000000000355, 3.000000000000000000, -7.050000000000000711 ) ) ;
#9875=AXIS2_PLACEMENT_3D ( 'NONE', #7376, #2542, #3692 ) ;
#9879=DIRECTION ( 'NONE',  ( 0.000000000000000000, 0.000000000000000000, 1.000000000000000000 ) ) ;
#9888=EDGE_CURVE ( 'NONE', #1838, #2349, #4237, .T. ) ;
#9908=VERTEX_POINT ( 'NONE', #5621 ) ;
#9924=AXIS2_PLACEMENT_3D ( 'NONE', #779, #8269, #907 ) ;
#9942=EDGE_CURVE ( 'NONE', #6484, #5272, #811, .T. ) ;
#9978=DIRECTION ( 'NONE',  ( -0.000000000000000000, -1.000000000000000000, -0.000000000000000000 ) ) ;
#9985=VERTEX_POINT ( 'NONE', #4730 ) ;
#9995=CARTESIAN_POINT ( 'NONE',  ( -5.999999999999991118, 3.000000000000000000, 27.00000000000000000 ) ) ;
#10004=ORIENTED_EDGE ( 'NONE', *, *, #9593, .T. ) ;
#10005=EDGE_CURVE ( 'NONE', #8988, #8770, #7149, .T. ) ;
#10007=AXIS2_PLACEMENT_3D ( 'NONE', #6754, #3381, #5712 ) ;
#10018=ORIENTED_EDGE ( 'NONE', *, *, #12580, .T. ) ;
#10036=EDGE_LOOP ( 'NONE', ( #6276, #12188 ) ) ;
#10040=EDGE_CURVE ( 'NONE', #1280, #12893, #9054, .T. ) ;
#10045=DIRECTION ( 'NONE',  ( 0.000000000000000000, 1.000000000000000000, 0.000000000000000000 ) ) ;
#10049=CARTESIAN_POINT ( 'NONE',  ( 6.000000000000008882, 3.000000000000000000, 27.00000000000000000 ) ) ;
#10071=VERTEX_POINT ( 'NONE', #6366 ) ;
#10083=DIRECTION ( 'NONE',  ( 0.000000000000000000, 0.000000000000000000, -1.000000000000000000 ) ) ;
#10089=CYLINDRICAL_SURFACE ( 'NONE', #1171, 2.999999999999999112 ) ;
#10097=VERTEX_POINT ( 'NONE', #11612 ) ;
#10115=ORIENTED_EDGE ( 'NONE', *, *, #3634, .T. ) ;
#10122=ORIENTED_EDGE ( 'NONE', *, *, #12741, .F. ) ;
#10150=DIRECTION ( 'NONE',  ( -0.000000000000000000, -1.000000000000000000, -0.000000000000000000 ) ) ;
#10159=FACE_OUTER_BOUND ( 'NONE', #10918, .T. ) ;
#10177=ADVANCED_FACE ( 'NONE', ( #9265 ), #2233, .F. ) ;
#10189=CIRCLE ( 'NONE', #3820, 8.500000000000000000 ) ;
#10193=VERTEX_POINT ( 'NONE', #6236 ) ;
#10203=AXIS2_PLACEMENT_3D ( 'NONE', #5177, #906, #13516 ) ;
#10212=VERTEX_POINT ( 'NONE', #10370 ) ;
#10216=ORIENTED_EDGE ( 'NONE', *, *, #11300, .T. ) ;
#10226=AXIS2_PLACEMENT_3D ( 'NONE', #9262, #13476, #12466 ) ;
#10239=EDGE_CURVE ( 'NONE', #4741, #4201, #2490, .T. ) ;
#10274=CARTESIAN_POINT ( 'NONE',  ( -8.222660081691577361, 3.000000000000000000, -8.549999999999998934 ) ) ;
#10278=EDGE_CURVE ( 'NONE', #2558, #5359, #10189, .T. ) ;
#10292=CARTESIAN_POINT ( 'NONE',  ( 20.00000000000000355, 0.000000000000000000, -14.92471123914604370 ) ) ;
#10293=DIRECTION ( 'NONE',  ( -0.000000000000000000, -1.000000000000000000, -0.000000000000000000 ) ) ;
#10334=AXIS2_PLACEMENT_3D ( 'NONE', #381, #1335, #11876 ) ;
#10336=AXIS2_PLACEMENT_3D ( 'NONE', #11453, #6092, #5251 ) ;
#10358=DIRECTION ( 'NONE',  ( -0.000000000000000000, -1.000000000000000000, -0.000000000000000000 ) ) ;
#10360=AXIS2_PLACEMENT_3D ( 'NONE', #8113, #1926, #5156 ) ;
#10362=ORIENTED_EDGE ( 'NONE', *, *, #3070, .F. ) ;
#10364=ORIENTED_EDGE ( 'NONE', *, *, #5729, .T. ) ;
#10365=CARTESIAN_POINT ( 'NONE',  ( 7.702138240596516638, 0.000000000000000000, -27.99999999999999289 ) ) ;
#10370=CARTESIAN_POINT ( 'NONE',  ( 19.44487669093179605, 0.000000000000000000, -16.66326752702930847 ) ) ;
#10376=DIRECTION ( 'NONE',  ( -1.261435711112880913E-16, -0.000000000000000000, -1.000000000000000000 ) ) ;
#10405=DIRECTION ( 'NONE',  ( 0.000000000000000000, 0.000000000000000000, 1.000000000000000000 ) ) ;
#10411=VECTOR ( 'NONE', #4275, 1000.000000000000000 ) ;
#10412=DIRECTION ( 'NONE',  ( 0.000000000000000000, 0.000000000000000000, 1.000000000000000000 ) ) ;
#10419=ORIENTED_EDGE ( 'NONE', *, *, #6813, .F. ) ;
#10420=AXIS2_PLACEMENT_3D ( 'NONE', #13122, #8973, #11260 ) ;
#10424=PLANE ( 'NONE',  #560 ) ;
#10441=DIRECTION ( 'NONE',  ( 0.000000000000000000, 0.000000000000000000, 1.000000000000000000 ) ) ;
#10442=VECTOR ( 'NONE', #7002, 1000.000000000000000 ) ;
#10448=CARTESIAN_POINT ( 'NONE',  ( 13.50000000000000355, 0.000000000000000000, -7.050000000000000711 ) ) ;
#10453=EDGE_CURVE ( 'NONE', #10888, #12681, #13053, .T. ) ;
#10454=FACE_OUTER_BOUND ( 'NONE', #9572, .T. ) ;
#10471=ORIENTED_EDGE ( 'NONE', *, *, #4253, .F. ) ;
#10479=DIRECTION ( 'NONE',  ( -0.000000000000000000, -1.000000000000000000, -0.000000000000000000 ) ) ;
#10482=CARTESIAN_POINT ( 'NONE',  ( 7.500000000000003553, 3.000000000000000000, 13.39999999999999858 ) ) ;
#10504=ORIENTED_EDGE ( 'NONE', *, *, #8537, .F. ) ;
#10514=ADVANCED_FACE ( 'NONE', ( #6288 ), #923, .F. ) ;
#10518=CARTESIAN_POINT ( 'NONE',  ( 13.50000000000000355, 3.000000000000000000, -7.050000000000000711 ) ) ;
#10539=DIRECTION ( 'NONE',  ( 0.000000000000000000, 0.000000000000000000, -1.000000000000000000 ) ) ;
#10548=DIRECTION ( 'NONE',  ( 0.000000000000000000, 0.000000000000000000, 1.000000000000000000 ) ) ;
#10552=VECTOR ( 'NONE', #9069, 1000.000000000000000 ) ;
#10562=CYLINDRICAL_SURFACE ( 'NONE', #1813, 1.499999999999997780 ) ;
#10578=DIRECTION ( 'NONE',  ( 0.000000000000000000, 0.000000000000000000, -1.000000000000000000 ) ) ;
#10600=DIRECTION ( 'NONE',  ( 0.000000000000000000, 0.000000000000000000, 1.000000000000000000 ) ) ;
#10628=( NAMED_UNIT ( * ) SI_UNIT ( $, .STERADIAN. ) SOLID_ANGLE_UNIT ( ) );
#10633=DIRECTION ( 'NONE',  ( 0.000000000000000000, 0.000000000000000000, 1.000000000000000000 ) ) ;
#10665=CARTESIAN_POINT ( 'NONE',  ( 13.50000000000000355, 3.000000000000000000, -5.550000000000001599 ) ) ;
#10677=EDGE_LOOP ( 'NONE', ( #7590, #3197, #4030, #11078 ) ) ;
#10678=( GEOMETRIC_REPRESENTATION_CONTEXT ( 3 ) GLOBAL_UNCERTAINTY_ASSIGNED_CONTEXT ( ( #1729 ) ) GLOBAL_UNIT_ASSIGNED_CONTEXT ( ( #103, #7456, #10628 ) ) REPRESENTATION_CONTEXT ( 'NONE', 'WORKASPACE' ) );
#10681=DIRECTION ( 'NONE',  ( -0.000000000000000000, -1.000000000000000000, -0.000000000000000000 ) ) ;
#10683=DIRECTION ( 'NONE',  ( 0.000000000000000000, 1.000000000000000000, 0.000000000000000000 ) ) ;
#10686=EDGE_CURVE ( 'NONE', #7585, #3491, #8746, .T. ) ;
#10693=CARTESIAN_POINT ( 'NONE',  ( 7.500000000000003553, 3.000000000000000000, 4.899999999999997691 ) ) ;
#10695=DIRECTION ( 'NONE',  ( -1.269138026879196405E-16, 0.000000000000000000, -1.000000000000000000 ) ) ;
#10696=CYLINDRICAL_SURFACE ( 'NONE', #9731, 1.500000000000001332 ) ;
#10709=ORIENTED_EDGE ( 'NONE', *, *, #3041, .F. ) ;
#10734=VERTEX_POINT ( 'NONE', #634 ) ;
#10743=CARTESIAN_POINT ( 'NONE',  ( 7.500000000000004441, 3.000000000000000000, 21.89999999999999858 ) ) ;
#10754=ORIENTED_EDGE ( 'NONE', *, *, #7588, .T. ) ;
#10772=FACE_OUTER_BOUND ( 'NONE', #12816, .T. ) ;
#10790=CARTESIAN_POINT ( 'NONE',  ( -5.999999999999991118, 0.000000000000000000, 25.50000000000000000 ) ) ;
#10800=DIRECTION ( 'NONE',  ( -0.000000000000000000, -1.000000000000000000, -0.000000000000000000 ) ) ;
#10810=ORIENTED_EDGE ( 'NONE', *, *, #3909, .F. ) ;
#10811=UNCERTAINTY_MEASURE_WITH_UNIT (LENGTH_MEASURE( 1.000000000000000082E-05 ), #11858, 'distance_accuracy_value', 'NONE');
#10820=SURFACE_SIDE_STYLE ('',( #9716 ) ) ;
#10823=DIRECTION ( 'NONE',  ( -1.000000000000000000, -0.000000000000000000, -0.000000000000000000 ) ) ;
#10824=DIRECTION ( 'NONE',  ( 0.000000000000000000, 1.000000000000000000, 0.000000000000000000 ) ) ;
#10831=ORIENTED_EDGE ( 'NONE', *, *, #3303, .T. ) ;
#10839=VECTOR ( 'NONE', #12895, 1000.000000000000000 ) ;
#10859=DIRECTION ( 'NONE',  ( 0.000000000000000000, 0.000000000000000000, 1.000000000000000000 ) ) ;
#10873=ORIENTED_EDGE ( 'NONE', *, *, #11479, .T. ) ;
#10876=ORIENTED_EDGE ( 'NONE', *, *, #2163, .F. ) ;
#10879=AXIS2_PLACEMENT_3D ( 'NONE', #889, #7021, #13425 ) ;
#10882=LINE ( 'NONE', #11084, #5814 ) ;
#10886=ORIENTED_EDGE ( 'NONE', *, *, #7136, .F. ) ;
#10888=VERTEX_POINT ( 'NONE', #975 ) ;
#10892=VERTEX_POINT ( 'NONE', #3095 ) ;
#10896=LINE ( 'NONE', #6971, #894 ) ;
#10900=DIRECTION ( 'NONE',  ( -0.6204948238377417935, -0.000000000000000000, 0.7842105416216806901 ) ) ;
#10906=ORIENTED_EDGE ( 'NONE', *, *, #8021, .T. ) ;
#10913=EDGE_CURVE ( 'NONE', #11282, #9985, #2282, .T. ) ;
#10918=EDGE_LOOP ( 'NONE', ( #7469, #1204, #867, #12921 ) ) ;
#10926=DIRECTION ( 'NONE',  ( 0.000000000000000000, 0.000000000000000000, 1.000000000000000000 ) ) ;
#10936=DIRECTION ( 'NONE',  ( 0.000000000000000000, 0.000000000000000000, -1.000000000000000000 ) ) ;
#10962=EDGE_CURVE ( 'NONE', #4201, #4741, #11965, .T. ) ;
#10969=ORIENTED_EDGE ( 'NONE', *, *, #13230, .F. ) ;
#10986=LINE ( 'NONE', #5958, #4033 ) ;
#10987=CARTESIAN_POINT ( 'NONE',  ( 7.500000000000003553, 0.000000000000000000, 13.39999999999999858 ) ) ;
#10989=AXIS2_PLACEMENT_3D ( 'NONE', #10448, #8496, #3205 ) ;
#10995=DIRECTION ( 'NONE',  ( -0.000000000000000000, -1.000000000000000000, -0.000000000000000000 ) ) ;
#10998=ORIENTED_EDGE ( 'NONE', *, *, #12268, .T. ) ;
#11009=CARTESIAN_POINT ( 'NONE',  ( -5.250000000000000000, 3.000000000000000000, -26.44078293894052578 ) ) ;
#11015=CARTESIAN_POINT ( 'NONE',  ( -8.352599575481690408, 3.000000000000000000, 30.99999999999999289 ) ) ;
#11024=DIRECTION ( 'NONE',  ( -1.000000000000000000, -0.000000000000000000, 1.055752450943286591E-16 ) ) ;
#11031=CIRCLE ( 'NONE', #4873, 2.999999999999999112 ) ;
#11047=CARTESIAN_POINT ( 'NONE',  ( 19.60942157306000766, 0.000000000000000000, 14.05941790610251374 ) ) ;
#11048=FACE_OUTER_BOUND ( 'NONE', #6014, .T. ) ;
#11057=EDGE_CURVE ( 'NONE', #5801, #3370, #9332, .T. ) ;
#11071=ORIENTED_EDGE ( 'NONE', *, *, #130, .T. ) ;
#11075=CARTESIAN_POINT ( 'NONE',  ( -13.28140389626389783, 0.000000000000000000, -1.567980996311402420 ) ) ;
#11078=ORIENTED_EDGE ( 'NONE', *, *, #13096, .T. ) ;
#11083=CIRCLE ( 'NONE', #8864, 1.500000000000001332 ) ;
#11084=CARTESIAN_POINT ( 'NONE',  ( -21.21140389626389577, 0.000000000000000000, -14.83930531255815133 ) ) ;
#11086=DIRECTION ( 'NONE',  ( 0.000000000000000000, 0.000000000000000000, -1.000000000000000000 ) ) ;
#11125=DIRECTION ( 'NONE',  ( 0.000000000000000000, 0.000000000000000000, 1.000000000000000000 ) ) ;
#11128=ORIENTED_EDGE ( 'NONE', *, *, #8948, .T. ) ;
#11133=EDGE_CURVE ( 'NONE', #7608, #8988, #7140, .T. ) ;
#11135=DIRECTION ( 'NONE',  ( 0.4933917819034832619, -0.000000000000000000, -0.8698071910200015910 ) ) ;
#11136=CARTESIAN_POINT ( 'NONE',  ( -13.28140389626389783, 3.000000000000000000, -1.567980996311402420 ) ) ;
#11138=ADVANCED_FACE ( 'NONE', ( #11845 ), #2404, .F. ) ;
#11162=DIRECTION ( 'NONE',  ( 0.000000000000000000, 0.000000000000000000, 1.000000000000000000 ) ) ;
#11163=EDGE_CURVE ( 'NONE', #5256, #1838, #10882, .T. ) ;
#11188=DIRECTION ( 'NONE',  ( 0.000000000000000000, -0.000000000000000000, -1.000000000000000000 ) ) ;
#11250=VERTEX_POINT ( 'NONE', #5699 ) ;
#11251=CARTESIAN_POINT ( 'NONE',  ( 5.250000000000000000, 3.000000000000000000, -27.94078293894052578 ) ) ;
#11257=VECTOR ( 'NONE', #5254, 1000.000000000000000 ) ;
#11260=DIRECTION ( 'NONE',  ( 0.000000000000000000, 0.000000000000000000, -1.000000000000000000 ) ) ;
#11272=DIRECTION ( 'NONE',  ( -0.000000000000000000, -1.000000000000000000, -0.000000000000000000 ) ) ;
#11275=AXIS2_PLACEMENT_3D ( 'NONE', #1191, #2418, #6490 ) ;
#11280=CARTESIAN_POINT ( 'NONE',  ( 7.500000000000003553, 3.000000000000000000, 13.39999999999999858 ) ) ;
#11282=VERTEX_POINT ( 'NONE', #11009 ) ;
#11283=VECTOR ( 'NONE', #8723, 1000.000000000000000 ) ;
#11300=EDGE_CURVE ( 'NONE', #10734, #12681, #8253, .T. ) ;
#11334=CARTESIAN_POINT ( 'NONE',  ( -5.250000000000000000, 0.000000000000000000, -27.94078293894052578 ) ) ;
#11352=CARTESIAN_POINT ( 'NONE',  ( -5.999999999999991118, 3.000000000000000000, 25.50000000000000000 ) ) ;
#11353=SHAPE_REPRESENTATION ( 'base-plate', ( #10007 ), #10678 ) ;
#11355=CYLINDRICAL_SURFACE ( 'NONE', #2034, 1.500000000000001332 ) ;
#11372=EDGE_CURVE ( 'NONE', #1409, #1736, #7362, .T. ) ;
#11378=DIRECTION ( 'NONE',  ( 0.000000000000000000, 0.000000000000000000, -1.000000000000000000 ) ) ;
#11382=ORIENTED_EDGE ( 'NONE', *, *, #4930, .F. ) ;
#11394=DIRECTION ( 'NONE',  ( -0.000000000000000000, -1.000000000000000000, -0.000000000000000000 ) ) ;
#11395=CARTESIAN_POINT ( 'NONE',  ( -10.15083332828461771, 3.000000000000000000, -29.86148447151320795 ) ) ;
#11400=ORIENTED_EDGE ( 'NONE', *, *, #92, .T. ) ;
#11401=LINE ( 'NONE', #9331, #3792 ) ;
#11407=DIRECTION ( 'NONE',  ( 0.000000000000000000, 0.000000000000000000, 1.000000000000000000 ) ) ;
#11415=EDGE_LOOP ( 'NONE', ( #2316, #2051, #12957, #5376 ) ) ;
#11418=CARTESIAN_POINT ( 'NONE',  ( -18.21140389626389222, 3.000000000000000000, 12.49772878833446299 ) ) ;
#11431=VECTOR ( 'NONE', #12536, 1000.000000000000000 ) ;
#11445=ORIENTED_EDGE ( 'NONE', *, *, #11163, .T. ) ;
#11450=DIRECTION ( 'NONE',  ( 0.000000000000000000, 0.000000000000000000, 1.000000000000000000 ) ) ;
#11453=CARTESIAN_POINT ( 'NONE',  ( 13.50000000000000355, 3.000000000000000000, -7.050000000000000711 ) ) ;
#11456=CARTESIAN_POINT ( 'NONE',  ( 13.50000000000000355, 3.000000000000000000, -7.050000000000000711 ) ) ;
#11479=EDGE_CURVE ( 'NONE', #732, #447, #3178, .T. ) ;
#11481=DIRECTION ( 'NONE',  ( 0.000000000000000000, 0.000000000000000000, -1.000000000000000000 ) ) ;
#11534=AXIS2_PLACEMENT_3D ( 'NONE', #10987, #1559, #9879 ) ;
#11542=ORIENTED_EDGE ( 'NONE', *, *, #9513, .T. ) ;
#11565=CIRCLE ( 'NONE', #4734, 1.500000000000001332 ) ;
#11577=VERTEX_POINT ( 'NONE', #6859 ) ;
#11586=DIRECTION ( 'NONE',  ( 0.000000000000000000, 1.000000000000000000, 0.000000000000000000 ) ) ;
#11594=EDGE_CURVE ( 'NONE', #2964, #5704, #457, .T. ) ;
#11596=FACE_OUTER_BOUND ( 'NONE', #7451, .T. ) ;
#11602=CARTESIAN_POINT ( 'NONE',  ( 10.14701493152832512, 3.000000000000000000, -29.73855628788322747 ) ) ;
#11604=ORIENTED_EDGE ( 'NONE', *, *, #6588, .F. ) ;
#11611=LINE ( 'NONE', #9466, #3176 ) ;
#11612=CARTESIAN_POINT ( 'NONE',  ( 5.250000000000000000, 0.000000000000000000, -29.44078293894052933 ) ) ;
#11621=DIRECTION ( 'NONE',  ( -0.000000000000000000, -1.000000000000000000, -0.000000000000000000 ) ) ;
#11633=ORIENTED_EDGE ( 'NONE', *, *, #5705, .F. ) ;
#11634=ORIENTED_EDGE ( 'NONE', *, *, #2752, .F. ) ;
#11639=VERTEX_POINT ( 'NONE', #12997 ) ;
#11647=ORIENTED_EDGE ( 'NONE', *, *, #5069, .F. ) ;
#11682=FACE_OUTER_BOUND ( 'NONE', #12725, .T. ) ;
#11693=CARTESIAN_POINT ( 'NONE',  ( 8.208497377870823897, 0.000000000000000000, -5.549999999999999822 ) ) ;
#11702=EDGE_CURVE ( 'NONE', #4625, #3023, #2529, .T. ) ;
#11708=CARTESIAN_POINT ( 'NONE',  ( -8.222660081691577361, 3.000000000000000000, -5.549999999999999822 ) ) ;
#11724=DIRECTION ( 'NONE',  ( 0.000000000000000000, 0.000000000000000000, -1.000000000000000000 ) ) ;
#11758=CIRCLE ( 'NONE', #9556, 2.999999999999999112 ) ;
#11819=EDGE_CURVE ( 'NONE', #375, #3649, #1398, .T. ) ;
#11824=EDGE_CURVE ( 'NONE', #4803, #2397, #12000, .T. ) ;
#11840=DIRECTION ( 'NONE',  ( 0.000000000000000000, 0.000000000000000000, 1.000000000000000000 ) ) ;
#11845=FACE_OUTER_BOUND ( 'NONE', #7849, .T. ) ;
#11850=CARTESIAN_POINT ( 'NONE',  ( -13.28140389626389783, 3.000000000000000000, 0.000000000000000000 ) ) ;
#11858=( LENGTH_UNIT ( ) NAMED_UNIT ( * ) SI_UNIT ( .MILLI., .METRE. ) );
#11859=CARTESIAN_POINT ( 'NONE',  ( 6.000000000000008882, 3.000000000000000000, 27.00000000000000000 ) ) ;
#11875=CARTESIAN_POINT ( 'NONE',  ( 13.50000000000000355, 0.000000000000000000, -7.050000000000000711 ) ) ;
#11876=DIRECTION ( 'NONE',  ( 0.000000000000000000, 0.000000000000000000, -1.000000000000000000 ) ) ;
#11884=CARTESIAN_POINT ( 'NONE',  ( 8.208497377870823897, 3.000000000000000000, -5.549999999999999822 ) ) ;
#11885=ORIENTED_EDGE ( 'NONE', *, *, #6175, .F. ) ;
#11887=CARTESIAN_POINT ( 'NONE',  ( -20.56403552112892896, 3.000000000000000000, -16.70078978407140013 ) ) ;
#11895=DIRECTION ( 'NONE',  ( 1.000000000000000000, 0.000000000000000000, 0.000000000000000000 ) ) ;
#11910=DIRECTION ( 'NONE',  ( 0.000000000000000000, 0.000000000000000000, -1.000000000000000000 ) ) ;
#11921=ORIENTED_EDGE ( 'NONE', *, *, #4128, .T. ) ;
#11935=ADVANCED_FACE ( 'NONE', ( #8133 ), #12360, .F. ) ;
#11952=DIRECTION ( 'NONE',  ( 0.000000000000000000, 1.000000000000000000, 0.000000000000000000 ) ) ;
#11954=CARTESIAN_POINT ( 'NONE',  ( 13.11311062740304401, 0.000000000000000000, -1.563624455674628377 ) ) ;
#11961=ORIENTED_EDGE ( 'NONE', *, *, #4321, .T. ) ;
#11965=CIRCLE ( 'NONE', #6031, 1.499999999999998668 ) ;
#11976=ADVANCED_FACE ( 'NONE', ( #2901 ), #1532, .F. ) ;
#12000=CIRCLE ( 'NONE', #5603, 1.500000000000001332 ) ;
#12005=SURFACE_STYLE_USAGE ( .BOTH. , #10820 ) ;
#12032=ORIENTED_EDGE ( 'NONE', *, *, #8027, .F. ) ;
#12034=ORIENTED_EDGE ( 'NONE', *, *, #10686, .T. ) ;
#12062=ORIENTED_EDGE ( 'NONE', *, *, #7177, .F. ) ;
#12065=CARTESIAN_POINT ( 'NONE',  ( 13.11311062740304401, 3.000000000000000000, -1.563624455674628377 ) ) ;
#12070=CARTESIAN_POINT ( 'NONE',  ( -8.222660081691577361, 0.000000000000000000, -5.549999999999999822 ) ) ;
#12088=EDGE_CURVE ( 'NONE', #3702, #8770, #13319, .T. ) ;
#12093=CARTESIAN_POINT ( 'NONE',  ( -7.798201703419555209, 3.000000000000000000, -30.99999999999999289 ) ) ;
#12106=AXIS2_PLACEMENT_3D ( 'NONE', #2634, #11394, #6286 ) ;
#12111=ORIENTED_EDGE ( 'NONE', *, *, #5313, .F. ) ;
#12114=CIRCLE ( 'NONE', #8140, 1.500000000000001332 ) ;
#12147=ORIENTED_EDGE ( 'NONE', *, *, #11057, .F. ) ;
#12151=ORIENTED_EDGE ( 'NONE', *, *, #1115, .F. ) ;
#12153=AXIS2_PLACEMENT_3D ( 'NONE', #8566, #1220, #8707 ) ;
#12156=ADVANCED_FACE ( 'NONE', ( #1106 ), #5301, .T. ) ;
#12164=FACE_BOUND ( 'NONE', #12648, .T. ) ;
#12166=DIRECTION ( 'NONE',  ( -0.000000000000000000, -1.000000000000000000, -0.000000000000000000 ) ) ;
#12167=APPLICATION_CONTEXT ( 'automotive_design' ) ;
#12174=ORIENTED_EDGE ( 'NONE', *, *, #12712, .T. ) ;
#12176=LINE ( 'NONE', #11887, #13524 ) ;
#12181=DIRECTION ( 'NONE',  ( -0.000000000000000000, -1.000000000000000000, -0.000000000000000000 ) ) ;
#12182=LINE ( 'NONE', #2655, #3521 ) ;
#12188=ORIENTED_EDGE ( 'NONE', *, *, #936, .F. ) ;
#12198=DIRECTION ( 'NONE',  ( 1.261435711112880913E-16, 0.000000000000000000, 1.000000000000000000 ) ) ;
#12209=DIRECTION ( 'NONE',  ( 0.000000000000000000, 0.000000000000000000, -1.000000000000000000 ) ) ;
#12232=CARTESIAN_POINT ( 'NONE',  ( -13.49999999999999645, 0.000000000000000000, -5.549999999999999822 ) ) ;
#12238=FACE_BOUND ( 'NONE', #13572, .T. ) ;
#12249=LINE ( 'NONE', #1700, #8854 ) ;
#12250=LINE ( 'NONE', #870, #10442 ) ;
#12258=FACE_OUTER_BOUND ( 'NONE', #9728, .T. ) ;
#12268=EDGE_CURVE ( 'NONE', #8454, #7299, #12889, .T. ) ;
#12279=ORIENTED_EDGE ( 'NONE', *, *, #7911, .F. ) ;
#12283=ORIENTED_EDGE ( 'NONE', *, *, #5650, .F. ) ;
#12308=ORIENTED_EDGE ( 'NONE', *, *, #12334, .F. ) ;
#12313=VERTEX_POINT ( 'NONE', #5573 ) ;
#12322=AXIS2_PLACEMENT_3D ( 'NONE', #4746, #2400, #8933 ) ;
#12330=AXIS2_PLACEMENT_3D ( 'NONE', #7624, #330, #2707 ) ;
#12334=EDGE_CURVE ( 'NONE', #833, #7638, #6803, .T. ) ;
#12338=CARTESIAN_POINT ( 'NONE',  ( -18.21140389626389222, 3.000000000000000000, 12.49772878833446299 ) ) ;
#12357=CIRCLE ( 'NONE', #12992, 2.999999999999999112 ) ;
#12359=DIRECTION ( 'NONE',  ( 1.000000000000000000, 0.000000000000000000, 0.000000000000000000 ) ) ;
#12360=PLANE ( 'NONE',  #3399 ) ;
#12361=ORIENTED_EDGE ( 'NONE', *, *, #7047, .F. ) ;
#12367=VECTOR ( 'NONE', #2122, 1000.000000000000000 ) ;
#12371=CARTESIAN_POINT ( 'NONE',  ( -20.74285254778206067, 0.000000000000000000, 14.10762559394868099 ) ) ;
#12383=ORIENTED_EDGE ( 'NONE', *, *, #5650, .T. ) ;
#12386=AXIS2_PLACEMENT_3D ( 'NONE', #12338, #13426, #8052 ) ;
#12404=AXIS2_PLACEMENT_3D ( 'NONE', #1363, #5561, #10936 ) ;
#12405=CIRCLE ( 'NONE', #1612, 1.500000000000001332 ) ;
#12406=AXIS2_PLACEMENT_3D ( 'NONE', #7982, #8942, #9003 ) ;
#12415=EDGE_CURVE ( 'NONE', #13469, #6080, #13094, .T. ) ;
#12421=ADVANCED_FACE ( 'NONE', ( #3852 ), #4813, .T. ) ;
#12425=ORIENTED_EDGE ( 'NONE', *, *, #31, .F. ) ;
#12427=CIRCLE ( 'NONE', #4044, 2.999999999999992450 ) ;
#12435=ORIENTED_EDGE ( 'NONE', *, *, #2150, .T. ) ;
#12437=ORIENTED_EDGE ( 'NONE', *, *, #5313, .T. ) ;
#12439=EDGE_LOOP ( 'NONE', ( #11604, #3707 ) ) ;
#12453=LINE ( 'NONE', #6096, #3540 ) ;
#12455=VECTOR ( 'NONE', #167, 1000.000000000000000 ) ;
#12461=VERTEX_POINT ( 'NONE', #3021 ) ;
#12466=DIRECTION ( 'NONE',  ( 0.5795187626277481518, 0.000000000000000000, 0.8149588969772670888 ) ) ;
#12511=CARTESIAN_POINT ( 'NONE',  ( -10.88404822699983576, 0.000000000000000000, 29.60989680561421622 ) ) ;
#12531=DIRECTION ( 'NONE',  ( 0.000000000000000000, 1.000000000000000000, 0.000000000000000000 ) ) ;
#12536=DIRECTION ( 'NONE',  ( -0.000000000000000000, -1.000000000000000000, -0.000000000000000000 ) ) ;
#12537=CARTESIAN_POINT ( 'NONE',  ( 13.50000000000000355, 3.000000000000000000, -8.549999999999998934 ) ) ;
#12552=VECTOR ( 'NONE', #12181, 1000.000000000000000 ) ;
#12560=ORIENTED_EDGE ( 'NONE', *, *, #7182, .F. ) ;
#12564=CARTESIAN_POINT ( 'NONE',  ( -5.250000000000000000, 0.000000000000000000, -29.44078293894052933 ) ) ;
#12580=EDGE_CURVE ( 'NONE', #8365, #8454, #9138, .T. ) ;
#12583=CARTESIAN_POINT ( 'NONE',  ( 7.500000000000003553, 3.000000000000000000, 1.399999999999998579 ) ) ;
#12626=VERTEX_POINT ( 'NONE', #11693 ) ;
#12627=ORIENTED_EDGE ( 'NONE', *, *, #9366, .F. ) ;
#12637=CARTESIAN_POINT ( 'NONE',  ( 8.252687871541629860, 3.000000000000000000, 31.00000000000000000 ) ) ;
#12648=EDGE_LOOP ( 'NONE', ( #12560, #2443, #10504, #7887, #10122, #3972, #6226, #10709 ) ) ;
#12674=CARTESIAN_POINT ( 'NONE',  ( -8.890701948131944476, 3.000000000000000000, 13.39999999999999858 ) ) ;
#12681=VERTEX_POINT ( 'NONE', #1289 ) ;
#12683=VERTEX_POINT ( 'NONE', #9686 ) ;
#12685=FACE_BOUND ( 'NONE', #9813, .T. ) ;
#12705=CARTESIAN_POINT ( 'NONE',  ( 13.50000000000000355, 3.000000000000000000, -7.050000000000000711 ) ) ;
#12712=EDGE_CURVE ( 'NONE', #2029, #10212, #6728, .T. ) ;
#12717=LINE ( 'NONE', #2314, #6187 ) ;
#12720=ORIENTED_EDGE ( 'NONE', *, *, #13266, .T. ) ;
#12725=EDGE_LOOP ( 'NONE', ( #2614, #5632, #7079, #9218 ) ) ;
#12732=DIRECTION ( 'NONE',  ( 0.000000000000000000, 1.000000000000000000, 0.000000000000000000 ) ) ;
#12737=EDGE_LOOP ( 'NONE', ( #2684, #13470, #12151, #12435 ) ) ;
#12741=EDGE_CURVE ( 'NONE', #1513, #5397, #8037, .T. ) ;
#12743=FACE_BOUND ( 'NONE', #6885, .T. ) ;
#12755=ORIENTED_EDGE ( 'NONE', *, *, #2752, .T. ) ;
#12759=DIRECTION ( 'NONE',  ( -0.000000000000000000, -1.000000000000000000, -0.000000000000000000 ) ) ;
#12761=FACE_OUTER_BOUND ( 'NONE', #13341, .T. ) ;
#12772=ADVANCED_FACE ( 'NONE', ( #12258 ), #7008, .F. ) ;
#12776=EDGE_LOOP ( 'NONE', ( #4276, #9661, #13371, #10969 ) ) ;
#12783=VECTOR ( 'NONE', #13147, 1000.000000000000000 ) ;
#12788=CARTESIAN_POINT ( 'NONE',  ( -20.56403552112892896, 3.000000000000000000, -16.70078978407140013 ) ) ;
#12792=ORIENTED_EDGE ( 'NONE', *, *, #12949, .F. ) ;
#12816=EDGE_LOOP ( 'NONE', ( #2408, #9816, #11961, #8275 ) ) ;
#12822=EDGE_CURVE ( 'NONE', #12313, #1251, #4862, .T. ) ;
#12823=VECTOR ( 'NONE', #9599, 1000.000000000000000 ) ;
#12850=DIRECTION ( 'NONE',  ( 0.000000000000000000, 0.000000000000000000, 1.000000000000000000 ) ) ;
#12857=EDGE_CURVE ( 'NONE', #7299, #8075, #2509, .T. ) ;
#12860=CYLINDRICAL_SURFACE ( 'NONE', #3999, 2.999999999999999112 ) ;
#12870=DIRECTION ( 'NONE',  ( 0.000000000000000000, 1.000000000000000000, -0.000000000000000000 ) ) ;
#12878=ORIENTED_EDGE ( 'NONE', *, *, #9888, .F. ) ;
#12884=AXIS2_PLACEMENT_3D ( 'NONE', #10049, #4681, #621 ) ;
#12887=CARTESIAN_POINT ( 'NONE',  ( -5.999999999999991118, 3.000000000000000000, 27.00000000000000000 ) ) ;
#12889=LINE ( 'NONE', #8667, #9360 ) ;
#12893=VERTEX_POINT ( 'NONE', #1919 ) ;
#12895=DIRECTION ( 'NONE',  ( 0.4933917819034832619, -0.000000000000000000, -0.8698071910200015910 ) ) ;
#12921=ORIENTED_EDGE ( 'NONE', *, *, #5705, .T. ) ;
#12930=CARTESIAN_POINT ( 'NONE',  ( -18.21140389626389222, 0.000000000000000000, 12.49772878833446299 ) ) ;
#12949=EDGE_CURVE ( 'NONE', #1736, #180, #12176, .T. ) ;
#12957=ORIENTED_EDGE ( 'NONE', *, *, #7184, .T. ) ;
#12959=SHAPE_REPRESENTATION_RELATIONSHIP ( 'NONE' , 'NONE' ,  #11353, #3745 ) ;
#12962=DIRECTION ( 'NONE',  ( -0.000000000000000000, -1.000000000000000000, -0.000000000000000000 ) ) ;
#12963=FACE_OUTER_BOUND ( 'NONE', #3296, .T. ) ;
#12967=ADVANCED_FACE ( 'NONE', ( #660 ), #5827, .F. ) ;
#12986=EDGE_CURVE ( 'NONE', #8240, #4834, #4713, .T. ) ;
#12988=ORIENTED_EDGE ( 'NONE', *, *, #12822, .T. ) ;
#12992=AXIS2_PLACEMENT_3D ( 'NONE', #105, #3246, #10633 ) ;
#12997=CARTESIAN_POINT ( 'NONE',  ( 20.00000000000000355, 3.000000000000000000, -14.92471123914604370 ) ) ;
#13016=ORIENTED_EDGE ( 'NONE', *, *, #5988, .T. ) ;
#13019=CLOSED_SHELL ( 'NONE', ( #1465, #10514, #7700, #1629, #3098, #11976, #9380, #3824, #6663, #6665, #2908, #1080, #11935, #1503, #13584, #1303, #10177, #7437, #2530, #133, #8593, #12156, #11138, #1881, #13151, #4978, #12967, #3059, #13543, #4082, #9396, #12421, #5063, #3683, #13489, #8183, #3733, #3613, #7825, #111, #6924, #12772, #3544, #1403, #118 ) ) ;
#13020=ORIENTED_EDGE ( 'NONE', *, *, #208, .F. ) ;
#13021=CARTESIAN_POINT ( 'NONE',  ( 19.60942157306000766, 3.000000000000000000, 14.05941790610251374 ) ) ;
#13031=VECTOR ( 'NONE', #11024, 1000.000000000000000 ) ;
#13035=DIRECTION ( 'NONE',  ( -0.000000000000000000, -1.000000000000000000, -0.000000000000000000 ) ) ;
#13037=ORIENTED_EDGE ( 'NONE', *, *, #3893, .F. ) ;
#13045=CARTESIAN_POINT ( 'NONE',  ( -13.49999999999999645, 0.000000000000000000, -7.049999999999998934 ) ) ;
#13053=CIRCLE ( 'NONE', #13285, 13.50000000000000178 ) ;
#13060=VECTOR ( 'NONE', #8555, 1000.000000000000000 ) ;
#13069=DIRECTION ( 'NONE',  ( 0.000000000000000000, 0.000000000000000000, -1.000000000000000000 ) ) ;
#13073=ORIENTED_EDGE ( 'NONE', *, *, #7184, .F. ) ;
#13080=ORIENTED_EDGE ( 'NONE', *, *, #12986, .T. ) ;
#13086=CIRCLE ( 'NONE', #8676, 1.500000000000001332 ) ;
#13089=DIRECTION ( 'NONE',  ( 0.000000000000000000, 0.000000000000000000, -1.000000000000000000 ) ) ;
#13094=CIRCLE ( 'NONE', #12884, 1.500000000000001332 ) ;
#13096=EDGE_CURVE ( 'NONE', #7606, #13159, #12250, .T. ) ;
#13115=DIRECTION ( 'NONE',  ( 0.000000000000000000, 1.000000000000000000, 0.000000000000000000 ) ) ;
#13122=CARTESIAN_POINT ( 'NONE',  ( -18.21140389626389577, 3.000000000000000000, -14.83930531255816376 ) ) ;
#13126=ORIENTED_EDGE ( 'NONE', *, *, #8822, .T. ) ;
#13147=DIRECTION ( 'NONE',  ( -0.000000000000000000, -1.000000000000000000, -0.000000000000000000 ) ) ;
#13151=ADVANCED_FACE ( 'NONE', ( #8230 ), #5061, .F. ) ;
#13154=ORIENTED_EDGE ( 'NONE', *, *, #7193, .T. ) ;
#13159=VERTEX_POINT ( 'NONE', #4163 ) ;
#13161=EDGE_CURVE ( 'NONE', #12893, #7299, #1422, .T. ) ;
#13166=LINE ( 'NONE', #12070, #13031 ) ;
#13183=DIRECTION ( 'NONE',  ( 0.000000000000000000, 1.000000000000000000, 0.000000000000000000 ) ) ;
#13184=FACE_BOUND ( 'NONE', #13307, .T. ) ;
#13185=EDGE_CURVE ( 'NONE', #5359, #8240, #11611, .T. ) ;
#13198=AXIS2_PLACEMENT_3D ( 'NONE', #3048, #3109, #5194 ) ;
#13207=CIRCLE ( 'NONE', #7919, 1.500000000000001332 ) ;
#13218=DIRECTION ( 'NONE',  ( -0.000000000000000000, -1.000000000000000000, -0.000000000000000000 ) ) ;
#13229=AXIS2_PLACEMENT_3D ( 'NONE', #7543, #9409, #10578 ) ;
#13230=EDGE_CURVE ( 'NONE', #12683, #10097, #996, .T. ) ;
#13239=DIRECTION ( 'NONE',  ( 0.7842105416216805791, -0.000000000000000000, 0.6204948238377419045 ) ) ;
#13260=CYLINDRICAL_SURFACE ( 'NONE', #9315, 13.50000000000000178 ) ;
#13266=EDGE_CURVE ( 'NONE', #7204, #2253, #4434, .T. ) ;
#13271=AXIS2_PLACEMENT_3D ( 'NONE', #1295, #148, #11840 ) ;
#13272=CARTESIAN_POINT ( 'NONE',  ( -13.28140389626389783, 0.000000000000000000, 13.39999999999999858 ) ) ;
#13273=AXIS2_PLACEMENT_3D ( 'NONE', #124, #2107, #6437 ) ;
#13274=EDGE_CURVE ( 'NONE', #11577, #1280, #8672, .T. ) ;
#13277=DIRECTION ( 'NONE',  ( 0.000000000000000000, 0.000000000000000000, 1.000000000000000000 ) ) ;
#13278=CARTESIAN_POINT ( 'NONE',  ( 11.65525440103098731, 3.000000000000000000, 2.142386537870793362 ) ) ;
#13282=ORIENTED_EDGE ( 'NONE', *, *, #12088, .F. ) ;
#13285=AXIS2_PLACEMENT_3D ( 'NONE', #8145, #4843, #1755 ) ;
#13296=ORIENTED_EDGE ( 'NONE', *, *, #4762, .F. ) ;
#13297=( LENGTH_UNIT ( ) NAMED_UNIT ( * ) SI_UNIT ( .MILLI., .METRE. ) );
#13304=VECTOR ( 'NONE', #5528, 1000.000000000000000 ) ;
#13307=EDGE_LOOP ( 'NONE', ( #361, #13037 ) ) ;
#13311=DIRECTION ( 'NONE',  ( 0.000000000000000000, 0.000000000000000000, -1.000000000000000000 ) ) ;
#13319=CIRCLE ( 'NONE', #7373, 1.500000000000001332 ) ;
#13336=DIRECTION ( 'NONE',  ( 0.000000000000000000, 0.000000000000000000, 1.000000000000000000 ) ) ;
#13341=EDGE_LOOP ( 'NONE', ( #6552, #9474, #11647, #8399 ) ) ;
#13352=DIRECTION ( 'NONE',  ( 0.000000000000000000, 0.000000000000000000, 1.000000000000000000 ) ) ;
#13371=ORIENTED_EDGE ( 'NONE', *, *, #8027, .T. ) ;
#13404=CARTESIAN_POINT ( 'NONE',  ( -8.352599575481690408, 0.000000000000000000, 28.00000000000000000 ) ) ;
#13417=DIRECTION ( 'NONE',  ( 0.000000000000000000, 0.000000000000000000, -1.000000000000000000 ) ) ;
#13425=DIRECTION ( 'NONE',  ( 0.000000000000000000, 0.000000000000000000, -1.000000000000000000 ) ) ;
#13426=DIRECTION ( 'NONE',  ( 0.000000000000000000, 1.000000000000000000, 0.000000000000000000 ) ) ;
#13434=ORIENTED_EDGE ( 'NONE', *, *, #6355, .T. ) ;
#13436=EDGE_LOOP ( 'NONE', ( #12755, #2629, #6827, #6194 ) ) ;
#13438=EDGE_CURVE ( 'NONE', #8770, #3702, #11565, .T. ) ;
#13447=DIRECTION ( 'NONE',  ( 0.000000000000000000, 0.000000000000000000, -1.000000000000000000 ) ) ;
#13450=ORIENTED_EDGE ( 'NONE', *, *, #4930, .T. ) ;
#13467=ORIENTED_EDGE ( 'NONE', *, *, #8537, .T. ) ;
#13468=DIRECTION ( 'NONE',  ( 0.000000000000000000, 0.000000000000000000, -1.000000000000000000 ) ) ;
#13469=VERTEX_POINT ( 'NONE', #4086 ) ;
#13470=ORIENTED_EDGE ( 'NONE', *, *, #8564, .F. ) ;
#13472=EDGE_LOOP ( 'NONE', ( #5483, #8693, #2696, #1364 ) ) ;
#13476=DIRECTION ( 'NONE',  ( -0.8149588969772670888, 0.000000000000000000, 0.5795187626277481518 ) ) ;
#13481=AXIS2_PLACEMENT_3D ( 'NONE', #9591, #6623, #3510 ) ;
#13489=ADVANCED_FACE ( 'NONE', ( #6089 ), #851, .T. ) ;
#13503=VECTOR ( 'NONE', #10995, 1000.000000000000000 ) ;
#13511=VECTOR ( 'NONE', #314, 1000.000000000000000 ) ;
#13516=DIRECTION ( 'NONE',  ( 0.000000000000000000, 0.000000000000000000, 1.000000000000000000 ) ) ;
#13524=VECTOR ( 'NONE', #1489, 1000.000000000000227 ) ;
#13543=ADVANCED_FACE ( 'NONE', ( #5446 ), #5192, .F. ) ;
#13546=ORIENTED_EDGE ( 'NONE', *, *, #9034, .F. ) ;
#13547=CARTESIAN_POINT ( 'NONE',  ( 19.44487669093179605, 3.000000000000000000, -16.66326752702930847 ) ) ;
#13572=EDGE_LOOP ( 'NONE', ( #10471, #8947 ) ) ;
#13581=EDGE_LOOP ( 'NONE', ( #6388, #2396 ) ) ;
#13583=CARTESIAN_POINT ( 'NONE',  ( 13.50000000000000355, 3.000000000000000000, -7.050000000000000711 ) ) ;
#13584=ADVANCED_FACE ( 'NONE', ( #7255 ), #10424, .F. ) ;
#13622=COLOUR_RGB('Dark Blue',0.08,0.2,0.34);
#13623=FILL_AREA_STYLE_COLOUR('',#13622);
#13624=FILL_AREA_STYLE('',(#13623));
#13625=SURFACE_STYLE_FILL_AREA(#13624);
#13626=SURFACE_SIDE_STYLE('',(#13625));
#13627=SURFACE_STYLE_USAGE(.BOTH.,#13626);
#13628=PRESENTATION_STYLE_ASSIGNMENT((#13627));
ENDSEC;
END-ISO-10303-21;
